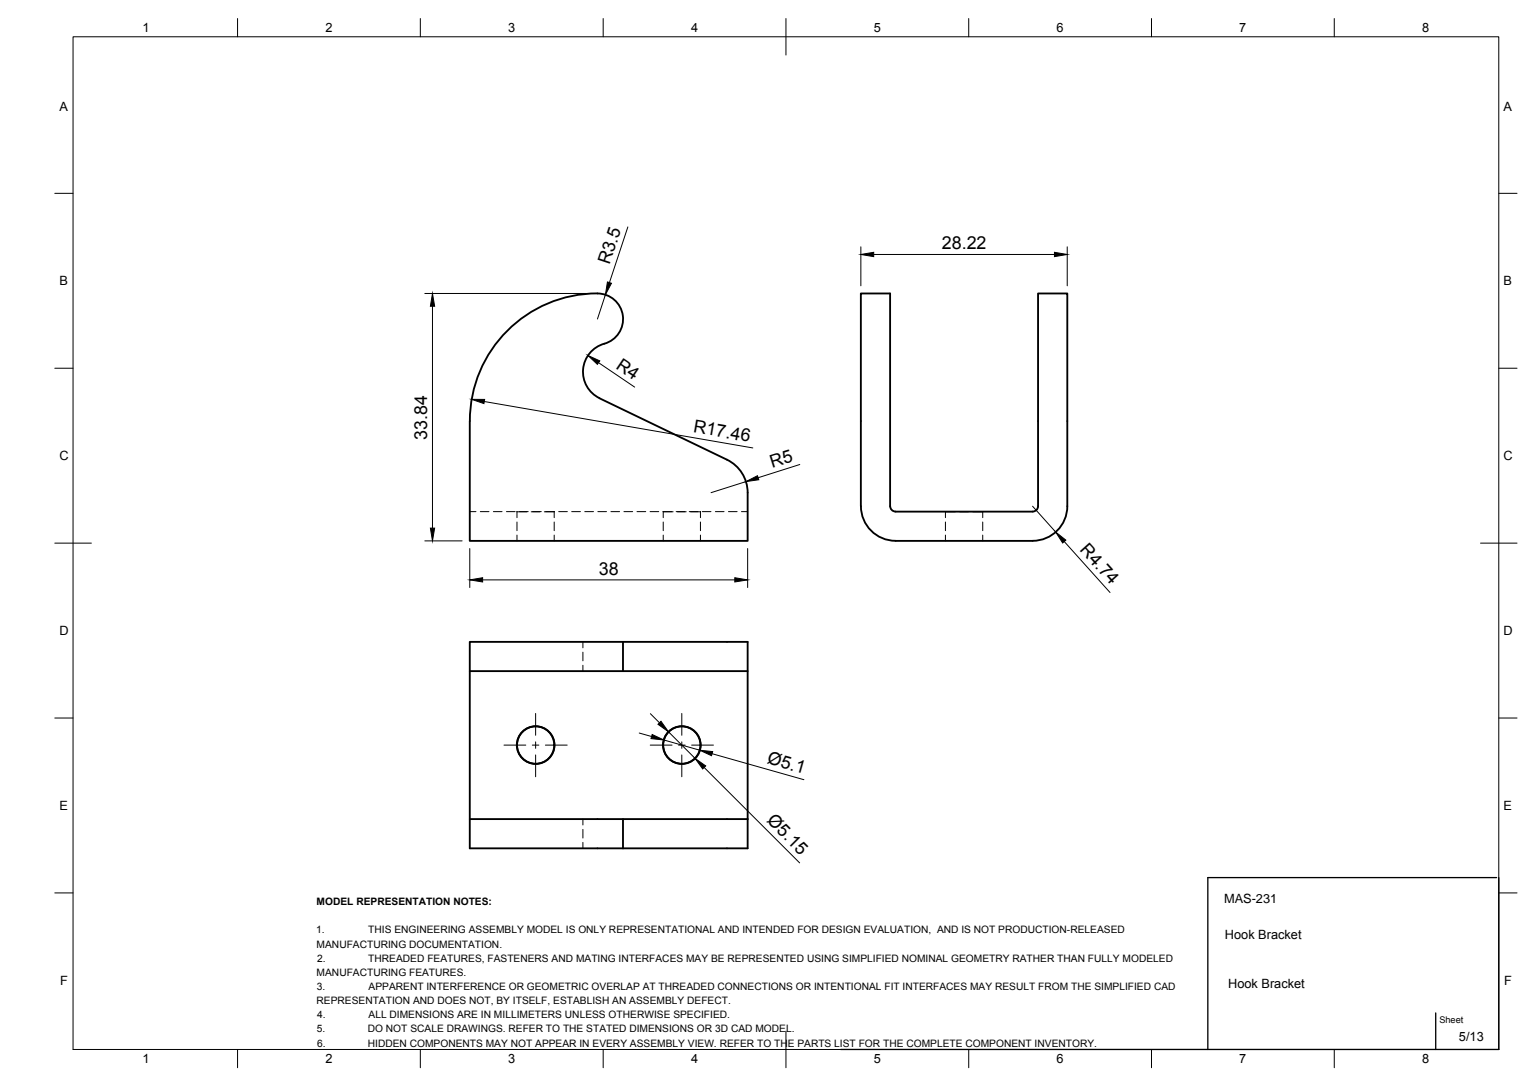
ISO-10303-21;
HEADER;
FILE_DESCRIPTION (('STEP AP214'),
    '1' );
FILE_NAME ( 'Hook Bracket.step', '2026-10-04T02:08:54', ( '' ), ( '' ), 'STEP AP214', 'Unspecified', '' );
FILE_SCHEMA (( 'AUTOMOTIVE_DESIGN' ));
ENDSEC;
DATA;
#98=ORIENTED_EDGE ( 'NONE', *, *, #40284, .T. ) ;
#119=EDGE_LOOP ( 'NONE', ( #9384, #25327, #26730, #11644 ) ) ;
#157=VERTEX_POINT ( 'NONE', #7543 ) ;
#241=ORIENTED_EDGE ( 'NONE', *, *, #39973, .T. ) ;
#254=EDGE_CURVE ( 'NONE', #18975, #21109, #11079, .T. ) ;
#326=AXIS2_PLACEMENT_3D ( 'NONE', #47306, #10657, #25265 ) ;
#395=AXIS2_PLACEMENT_3D ( 'NONE', #5918, #35170, #24842 ) ;
#397=CARTESIAN_POINT ( 'NONE',  ( -0.5555748031496061667, 0.1864803149606364951, -0.7480314960629921295 ) ) ;
#449=CIRCLE ( 'NONE', #39490, 0.02900000000000001882 ) ;
#498=CARTESIAN_POINT ( 'NONE',  ( 0.5555748031496077211, 2.215965818540671970E-15, 0.7480314960629921295 ) ) ;
#504=CIRCLE ( 'NONE', #41823, 0.1003937007874011050 ) ;
#509=ORIENTED_EDGE ( 'NONE', *, *, #3081, .F. ) ;
#538=CARTESIAN_POINT ( 'NONE',  ( -0.5555748031496058337, 0.2597269656108975311, 0.7480314960629921295 ) ) ;
#660=AXIS2_PLACEMENT_3D ( 'NONE', #17202, #46421, #20086 ) ;
#686=EDGE_CURVE ( 'NONE', #23816, #39475, #34433, .T. ) ;
#789=DIRECTION ( 'NONE',  ( -0.000000000000000000, 1.000000000000000000, -0.000000000000000000 ) ) ;
#867=CARTESIAN_POINT ( 'NONE',  ( 0.5555748031496089423, 0.3833307086614172743, 0.7480314960629921295 ) ) ;
#931=ORIENTED_EDGE ( 'NONE', *, *, #9551, .T. ) ;
#1004=VERTEX_POINT ( 'NONE', #1577 ) ;
#1044=CARTESIAN_POINT ( 'NONE',  ( 1.739107093083948175E-16, 0.1574803149606340824, 0.2923228346456709370 ) ) ;
#1068=DIRECTION ( 'NONE',  ( 1.541976423090495042E-15, 0.4344452574044150306, -0.9006982393225888561 ) ) ;
#1160=ORIENTED_EDGE ( 'NONE', *, *, #40875, .T. ) ;
#1198=EDGE_CURVE ( 'NONE', #23361, #25294, #34801, .T. ) ;
#1237=ORIENTED_EDGE ( 'NONE', *, *, #25095, .T. ) ;
#1310=DIRECTION ( 'NONE',  ( -1.000000000000000000, 3.469446951953613794E-15, 0.000000000000000000 ) ) ;
#1348=DIRECTION ( 'NONE',  ( 1.000000000000000000, -3.469446951953613794E-15, -0.000000000000000000 ) ) ;
#1499=CARTESIAN_POINT ( 'NONE',  ( -0.3980944881889741382, 0.7681739484881660029, -0.04983111751016756213 ) ) ;
#1514=FACE_OUTER_BOUND ( 'NONE', #43262, .T. ) ;
#1557=DIRECTION ( 'NONE',  ( 1.000000000000000000, -3.469446951953613794E-15, -0.000000000000000000 ) ) ;
#1577=CARTESIAN_POINT ( 'NONE',  ( 1.614954907737318939E-16, 0.1574803149606340824, 0.4950787401574787139 ) ) ;
#1587=DIRECTION ( 'NONE',  ( 0.000000000000000000, -1.000000000000000000, 0.000000000000000000 ) ) ;
#1618=CARTESIAN_POINT ( 'NONE',  ( -7.957671378281915615E-17, 0.1574803149606340824, -0.2923228346456709370 ) ) ;
#1725=CARTESIAN_POINT ( 'NONE',  ( 0.3980944881889779130, 0.4370297686271517601, 0.6367018223237037589 ) ) ;
#1755=ORIENTED_EDGE ( 'NONE', *, *, #21966, .F. ) ;
#1809=EDGE_CURVE ( 'NONE', #39475, #34571, #39007, .T. ) ;
#1956=EDGE_LOOP ( 'NONE', ( #15134, #37598, #45628, #21040 ) ) ;
#1983=DIMENSIONAL_EXPONENTS ( 1.000000000000000000, 0.000000000000000000, 0.000000000000000000, 0.000000000000000000, 0.000000000000000000, 0.000000000000000000, 0.000000000000000000 ) ;
#2019=VERTEX_POINT ( 'NONE', #7328 ) ;
#2094=VECTOR ( 'NONE', #47331, 39.37007874015748854 ) ;
#2109=EDGE_CURVE ( 'NONE', #33977, #31956, #23129, .T. ) ;
#2130=ORIENTED_EDGE ( 'NONE', *, *, #32542, .F. ) ;
#2161=VECTOR ( 'NONE', #24206, 39.37007874015748143 ) ;
#2318=ADVANCED_FACE ( 'NONE', ( #29029 ), #46707, .T. ) ;
#2362=LINE ( 'NONE', #45498, #19120 ) ;
#2457=LINE ( 'NONE', #17083, #4486 ) ;
#2474=CARTESIAN_POINT ( 'NONE',  ( 0.3690944881889770546, 0.1574803149606328057, 0.7480314960629921295 ) ) ;
#2489=CYLINDRICAL_SURFACE ( 'NONE', #43547, 0.1377952755905521298 ) ;
#2593=AXIS2_PLACEMENT_3D ( 'NONE', #22968, #30429, #44981 ) ;
#2608=CARTESIAN_POINT ( 'NONE',  ( 0.5555748031496109407, 0.9100161909011688088, 0.01858545845903165558 ) ) ;
#2676=AXIS2_PLACEMENT_3D ( 'NONE', #36439, #10566, #40228 ) ;
#2701=FACE_OUTER_BOUND ( 'NONE', #16952, .T. ) ;
#2719=DIRECTION ( 'NONE',  ( -3.469446951953590129E-15, -1.000000000000000000, 0.000000000000000000 ) ) ;
#2727=FACE_OUTER_BOUND ( 'NONE', #31753, .T. ) ;
#2790=ORIENTED_EDGE ( 'NONE', *, *, #43590, .F. ) ;
#2886=ORIENTED_EDGE ( 'NONE', *, *, #14250, .T. ) ;
#2896=CARTESIAN_POINT ( 'NONE',  ( 0.5555748031496123840, 1.332209862199691397, -0.06082000038405670217 ) ) ;
#2949=DIRECTION ( 'NONE',  ( -0.000000000000000000, 1.000000000000000000, -0.000000000000000000 ) ) ;
#2984=EDGE_LOOP ( 'NONE', ( #4268, #8274, #16882, #28951, #15427, #2790, #46729, #33220 ) ) ;
#2993=EDGE_LOOP ( 'NONE', ( #6858, #21214, #41669, #27403 ) ) ;
#3042=CYLINDRICAL_SURFACE ( 'NONE', #26195, 0.1574803149606291142 ) ;
#3075=DIRECTION ( 'NONE',  ( 3.469446951953613794E-15, 1.000000000000000000, 0.000000000000000000 ) ) ;
#3081=EDGE_CURVE ( 'NONE', #34571, #38848, #8006, .T. ) ;
#3137=ORIENTED_EDGE ( 'NONE', *, *, #14250, .F. ) ;
#3165=VERTEX_POINT ( 'NONE', #10746 ) ;
#3205=FACE_OUTER_BOUND ( 'NONE', #16925, .T. ) ;
#3330=LINE ( 'NONE', #32591, #23506 ) ;
#3413=DIRECTION ( 'NONE',  ( 0.000000000000000000, 0.000000000000000000, -1.000000000000000000 ) ) ;
#3478=CARTESIAN_POINT ( 'NONE',  ( -0.5555748031496040573, 0.7681739484881665581, -0.04983111751016756213 ) ) ;
#3650=CARTESIAN_POINT ( 'NONE',  ( -0.3690944881889761664, 0.1574803149606353592, -0.7480314960629921295 ) ) ;
#3686=EDGE_CURVE ( 'NONE', #1004, #10953, #29361, .T. ) ;
#3744=AXIS2_PLACEMENT_3D ( 'NONE', #44263, #36406, #11461 ) ;
#3773=AXIS2_PLACEMENT_3D ( 'NONE', #35805, #2949, #32229 ) ;
#3778=VECTOR ( 'NONE', #30865, 39.37007874015748143 ) ;
#3862=MANIFOLD_SOLID_BREP ( 'Hook Bracket', #17070 ) ;
#3897=VECTOR ( 'NONE', #44937, 39.37007874015748854 ) ;
#3983=ADVANCED_FACE ( 'NONE', ( #13018 ), #33958, .T. ) ;
#4077=VERTEX_POINT ( 'NONE', #5814 ) ;
#4089=VECTOR ( 'NONE', #22486, 39.37007874015748143 ) ;
#4198=LINE ( 'NONE', #30373, #20248 ) ;
#4268=ORIENTED_EDGE ( 'NONE', *, *, #43106, .F. ) ;
#4318=CARTESIAN_POINT ( 'NONE',  ( 1.614954907737318939E-16, 0.1574803149606340824, 0.3937007874015748254 ) ) ;
#4360=ORIENTED_EDGE ( 'NONE', *, *, #40924, .F. ) ;
#4390=AXIS2_PLACEMENT_3D ( 'NONE', #10675, #40108, #14018 ) ;
#4486=VECTOR ( 'NONE', #16161, 39.37007874015748143 ) ;
#4561=ORIENTED_EDGE ( 'NONE', *, *, #23328, .T. ) ;
#4584=ORIENTED_EDGE ( 'NONE', *, *, #32997, .F. ) ;
#4633=AXIS2_PLACEMENT_3D ( 'NONE', #24573, #6345, #46368 ) ;
#4691=ADVANCED_FACE ( 'NONE', ( #21545, #20835, #17017 ), #27840, .T. ) ;
#4789=CIRCLE ( 'NONE', #46111, 0.1574803149606301966 ) ;
#4839=FACE_OUTER_BOUND ( 'NONE', #33641, .T. ) ;
#4908=FACE_OUTER_BOUND ( 'NONE', #46312, .T. ) ;
#4919=VECTOR ( 'NONE', #1557, 39.37007874015748143 ) ;
#4975=EDGE_CURVE ( 'NONE', #11301, #39475, #11250, .T. ) ;
#5022=AXIS2_PLACEMENT_3D ( 'NONE', #20568, #24186, #12707 ) ;
#5025=DIRECTION ( 'NONE',  ( -3.469446951953613794E-15, -1.000000000000000000, 0.000000000000000000 ) ) ;
#5134=EDGE_LOOP ( 'NONE', ( #14252, #38748, #44441, #32739, #28557, #35520, #1237, #38379, #3137, #241, #10330, #17989 ) ) ;
#5307=AXIS2_PLACEMENT_3D ( 'NONE', #24089, #24779, #39377 ) ;
#5350=FACE_OUTER_BOUND ( 'NONE', #46134, .T. ) ;
#5405=FACE_BOUND ( 'NONE', #26025, .T. ) ;
#5450=ORIENTED_EDGE ( 'NONE', *, *, #32997, .T. ) ;
#5466=ORIENTED_EDGE ( 'NONE', *, *, #16551, .T. ) ;
#5487=VECTOR ( 'NONE', #17364, 39.37007874015748854 ) ;
#5632=ORIENTED_EDGE ( 'NONE', *, *, #3686, .F. ) ;
#5727=UNCERTAINTY_MEASURE_WITH_UNIT (LENGTH_MEASURE( 1.000000000000000082E-05 ), #6167, 'distance_accuracy_value', 'NONE') ;
#5755=AXIS2_PLACEMENT_3D ( 'NONE', #8382, #41424, #22289 ) ;
#5756=ADVANCED_FACE ( 'NONE', ( #12240 ), #12007, .T. ) ;
#5783=DIRECTION ( 'NONE',  ( 0.000000000000000000, 0.7071067811865965336, 0.7071067811864983899 ) ) ;
#5814=CARTESIAN_POINT ( 'NONE',  ( 0.5555748031496103856, 0.7681739484881628943, -0.04983111751016747887 ) ) ;
#5816=CIRCLE ( 'NONE', #35657, 0.6872114956789353579 ) ;
#5832=DIRECTION ( 'NONE',  ( 3.469446951953626022E-15, 1.000000000000000000, 0.000000000000000000 ) ) ;
#5918=CARTESIAN_POINT ( 'NONE',  ( -0.3690944881889761109, 0.1864803149606353017, 0.7480314960629921295 ) ) ;
#5990=CARTESIAN_POINT ( 'NONE',  ( -0.5555748031496045014, 0.6449983665207589256, -0.7480314960629921295 ) ) ;
#5993=VERTEX_POINT ( 'NONE', #29714 ) ;
#6018=ORIENTED_EDGE ( 'NONE', *, *, #41186, .F. ) ;
#6167=( CONVERSION_BASED_UNIT ( 'INCH', #39466 ) LENGTH_UNIT ( ) NAMED_UNIT ( #22776 ) ) ;
#6188=AXIS2_PLACEMENT_3D ( 'NONE', #9502, #46136, #27264 ) ;
#6251=ORIENTED_EDGE ( 'NONE', *, *, #19100, .T. ) ;
#6325=CARTESIAN_POINT ( 'NONE',  ( 0.3980944881889795228, 0.9100161909011693639, 0.01858545845903165558 ) ) ;
#6345=DIRECTION ( 'NONE',  ( -3.469446951953613794E-15, -1.000000000000000000, 0.000000000000000000 ) ) ;
#6347=CARTESIAN_POINT ( 'NONE',  ( 0.3690944881889778317, 2.862949378880179425E-15, 0.7480314960629921295 ) ) ;
#6355=CARTESIAN_POINT ( 'NONE',  ( -0.3690944881889761109, 0.1864803149606354127, 0.7480314960629921295 ) ) ;
#6360=ORIENTED_EDGE ( 'NONE', *, *, #11275, .F. ) ;
#6368=ADVANCED_FACE ( 'NONE', ( #4908 ), #46344, .F. ) ;
#6376=CARTESIAN_POINT ( 'NONE',  ( 1.737901732061166719E-16, 0.1564960629921311464, 0.2933070866141737065 ) ) ;
#6390=PRODUCT_DEFINITION ( 'UNKNOWN', '', #25524, #46091 ) ;
#6407=CARTESIAN_POINT ( 'NONE',  ( 0.5555748031496109407, 0.9100161909011688088, 0.01858545845903165558 ) ) ;
#6460=DIRECTION ( 'NONE',  ( 3.385139170096243171E-15, 1.000000000000000000, -0.000000000000000000 ) ) ;
#6558=CIRCLE ( 'NONE', #5022, 0.1003937007874011050 ) ;
#6641=FILL_AREA_STYLE_COLOUR ( '', #45353 ) ;
#6647=ORIENTED_EDGE ( 'NONE', *, *, #1809, .F. ) ;
#6682=DIRECTION ( 'NONE',  ( -3.469446951953613794E-15, -1.000000000000000000, -3.652049423109077687E-16 ) ) ;
#6742=( NAMED_UNIT ( * ) PLANE_ANGLE_UNIT ( ) SI_UNIT ( $, .RADIAN. ) ) ;
#6852=AXIS2_PLACEMENT_3D ( 'NONE', #10460, #31568, #14289 ) ;
#6858=ORIENTED_EDGE ( 'NONE', *, *, #12795, .F. ) ;
#6910=DIRECTION ( 'NONE',  ( 1.000000000000000000, -3.469446951953625233E-15, -0.000000000000000000 ) ) ;
#6936=EDGE_CURVE ( 'NONE', #13381, #27058, #4198, .T. ) ;
#6946=VECTOR ( 'NONE', #24006, 39.37007874015748143 ) ;
#7158=CARTESIAN_POINT ( 'NONE',  ( 0.5555748031496118289, 1.194414586609139128, -0.06082000038405787484 ) ) ;
#7197=VECTOR ( 'NONE', #26346, 39.37007874015748143 ) ;
#7244=FACE_OUTER_BOUND ( 'NONE', #5134, .T. ) ;
#7309=DIRECTION ( 'NONE',  ( -3.494233027178502331E-15, -1.000000000000000000, -0.000000000000000000 ) ) ;
#7328=CARTESIAN_POINT ( 'NONE',  ( -0.3690944881889767215, 5.970426471673286898E-15, -0.7480314960629921295 ) ) ;
#7332=ORIENTED_EDGE ( 'NONE', *, *, #16551, .F. ) ;
#7393=FACE_OUTER_BOUND ( 'NONE', #39319, .T. ) ;
#7416=ADVANCED_FACE ( 'NONE', ( #3205 ), #43453, .T. ) ;
#7428=ORIENTED_EDGE ( 'NONE', *, *, #45869, .F. ) ;
#7447=ORIENTED_EDGE ( 'NONE', *, *, #11487, .T. ) ;
#7543=CARTESIAN_POINT ( 'NONE',  ( 0.5555748031496099415, 0.6449983665207553729, -0.7480314960629920185 ) ) ;
#7566=ORIENTED_EDGE ( 'NONE', *, *, #9639, .F. ) ;
#7618=EDGE_CURVE ( 'NONE', #31956, #27577, #33425, .T. ) ;
#7621=ORIENTED_EDGE ( 'NONE', *, *, #13429, .T. ) ;
#7636=ORIENTED_EDGE ( 'NONE', *, *, #39035, .F. ) ;
#7689=SHAPE_REPRESENTATION_RELATIONSHIP ( 'NONE' , 'NONE' ,  #11151, #38737 ) ;
#7744=VERTEX_POINT ( 'NONE', #37865 ) ;
#7760=AXIS2_PLACEMENT_3D ( 'NONE', #42762, #35155, #1587 ) ;
#7773=ORIENTED_EDGE ( 'NONE', *, *, #43106, .T. ) ;
#7870=DIRECTION ( 'NONE',  ( -0.000000000000000000, 1.000000000000000000, -0.000000000000000000 ) ) ;
#7887=ORIENTED_EDGE ( 'NONE', *, *, #30299, .F. ) ;
#7975=AXIS2_PLACEMENT_3D ( 'NONE', #31654, #6682, #13888 ) ;
#7999=VECTOR ( 'NONE', #10189, 39.37007874015748143 ) ;
#8006=LINE ( 'NONE', #11627, #22275 ) ;
#8107=CARTESIAN_POINT ( 'NONE',  ( 0.5555748031496077211, 2.215965818540671970E-15, 0.7480314960629921295 ) ) ;
#8274=ORIENTED_EDGE ( 'NONE', *, *, #16350, .T. ) ;
#8355=CARTESIAN_POINT ( 'NONE',  ( -0.5555748031496021699, 1.332209862199694284, -0.06082000038405668829 ) ) ;
#8382=CARTESIAN_POINT ( 'NONE',  ( -0.3690944881889761109, 0.1864803149606356070, -0.06082000038405686176 ) ) ;
#8408=CARTESIAN_POINT ( 'NONE',  ( -6.728203135043436585E-17, -8.878505979408855953E-16, -0.4940944881889759444 ) ) ;
#8483=ORIENTED_EDGE ( 'NONE', *, *, #21818, .T. ) ;
#8491=CARTESIAN_POINT ( 'NONE',  ( -0.3980944881889759146, 0.2597269656108969760, 0.5511811023622046335 ) ) ;
#8503=ORIENTED_EDGE ( 'NONE', *, *, #30299, .T. ) ;
#8510=ORIENTED_EDGE ( 'NONE', *, *, #37835, .T. ) ;
#8584=APPLICATION_CONTEXT ( 'automotive_design' ) ;
#8604=ADVANCED_FACE ( 'NONE', ( #30707 ), #27119, .F. ) ;
#8676=VECTOR ( 'NONE', #6460, 39.37007874015748143 ) ;
#8731=CARTESIAN_POINT ( 'NONE',  ( 0.5555748031496083872, 0.1864803149606326926, -0.7480314960629921295 ) ) ;
#8737=CARTESIAN_POINT ( 'NONE',  ( -0.3980944881889755260, 0.3833307086614208270, 0.7480314960629921295 ) ) ;
#8832=DIRECTION ( 'NONE',  ( -3.469446951953613794E-15, -1.000000000000000000, 0.000000000000000000 ) ) ;
#8892=ORIENTED_EDGE ( 'NONE', *, *, #30656, .T. ) ;
#8924=DIRECTION ( 'NONE',  ( 0.000000000000000000, 1.000000000000000000, 0.000000000000000000 ) ) ;
#9004=CARTESIAN_POINT ( 'NONE',  ( -0.5555748031496040573, 0.7681739484881661140, -0.04983111751016786051 ) ) ;
#9056=CARTESIAN_POINT ( 'NONE',  ( -0.5555748031496045014, 0.6449983665207589256, -0.06082000038405668829 ) ) ;
#9100=EDGE_CURVE ( 'NONE', #14069, #33762, #27232, .T. ) ;
#9272=CYLINDRICAL_SURFACE ( 'NONE', #7760, 0.1864803149606299171 ) ;
#9280=ORIENTED_EDGE ( 'NONE', *, *, #28375, .F. ) ;
#9338=ORIENTED_EDGE ( 'NONE', *, *, #14169, .T. ) ;
#9384=ORIENTED_EDGE ( 'NONE', *, *, #43378, .T. ) ;
#9400=AXIS2_PLACEMENT_3D ( 'NONE', #4318, #8832, #12694 ) ;
#9464=VERTEX_POINT ( 'NONE', #16370 ) ;
#9479=VERTEX_POINT ( 'NONE', #1725 ) ;
#9502=CARTESIAN_POINT ( 'NONE',  ( -0.3980944881889745268, 0.6449983665207583705, -0.06082000038405668829 ) ) ;
#9523=DIRECTION ( 'NONE',  ( 1.000000000000000000, -3.469446951953614189E-15, -0.000000000000000000 ) ) ;
#9551=EDGE_CURVE ( 'NONE', #19046, #2019, #3330, .T. ) ;
#9554=SURFACE_STYLE_FILL_AREA ( #28238 ) ;
#9587=LINE ( 'NONE', #9824, #2161 ) ;
#9628=DIRECTION ( 'NONE',  ( 3.469446951953608272E-15, 1.000000000000000000, 0.000000000000000000 ) ) ;
#9639=EDGE_CURVE ( 'NONE', #35496, #36366, #504, .T. ) ;
#9692=FACE_OUTER_BOUND ( 'NONE', #1956, .T. ) ;
#9714=CYLINDRICAL_SURFACE ( 'NONE', #17689, 0.02900000000000001882 ) ;
#9738=ORIENTED_EDGE ( 'NONE', *, *, #31992, .T. ) ;
#9757=ADVANCED_FACE ( 'NONE', ( #4839 ), #12039, .F. ) ;
#9807=CIRCLE ( 'NONE', #4390, 0.1003937007874011050 ) ;
#9824=CARTESIAN_POINT ( 'NONE',  ( 1.737901732061166719E-16, 0.1574803149606340824, 0.2933070866141737065 ) ) ;
#9915=VECTOR ( 'NONE', #5783, 39.37007874015748854 ) ;
#9937=DIRECTION ( 'NONE',  ( -1.000000000000000000, 3.469446951953614189E-15, 0.000000000000000000 ) ) ;
#9969=ADVANCED_FACE ( 'NONE', ( #2701 ), #13973, .F. ) ;
#10002=VECTOR ( 'NONE', #1068, 39.37007874015748854 ) ;
#10051=DIRECTION ( 'NONE',  ( 1.000000000000000000, 0.000000000000000000, 0.000000000000000000 ) ) ;
#10104=AXIS2_PLACEMENT_3D ( 'NONE', #15674, #44861, #30080 ) ;
#10189=DIRECTION ( 'NONE',  ( -1.000000000000000000, 3.469446951953613794E-15, 0.000000000000000000 ) ) ;
#10222=VERTEX_POINT ( 'NONE', #38556 ) ;
#10257=CARTESIAN_POINT ( 'NONE',  ( -0.3690944881889761109, 0.1864803149606358568, -0.7480314960629921295 ) ) ;
#10301=ORIENTED_EDGE ( 'NONE', *, *, #45389, .F. ) ;
#10330=ORIENTED_EDGE ( 'NONE', *, *, #30656, .F. ) ;
#10333=ORIENTED_EDGE ( 'NONE', *, *, #16196, .F. ) ;
#10337=CONICAL_SURFACE ( 'NONE', #34066, 0.1003937007874011050, 0.7853981633973787790 ) ;
#10460=CARTESIAN_POINT ( 'NONE',  ( 0.3690944881889771101, 0.1864803149606328037, -0.7480314960629921295 ) ) ;
#10480=ORIENTED_EDGE ( 'NONE', *, *, #19100, .F. ) ;
#10566=DIRECTION ( 'NONE',  ( -0.000000000000000000, 1.000000000000000000, -0.000000000000000000 ) ) ;
#10657=DIRECTION ( 'NONE',  ( -1.000000000000000000, 3.469446951953614189E-15, 0.000000000000000000 ) ) ;
#10667=CARTESIAN_POINT ( 'NONE',  ( 0.3980944881889786346, 0.6449983665207558170, -0.06082000038405668829 ) ) ;
#10675=CARTESIAN_POINT ( 'NONE',  ( 1.614954907737318939E-16, 0.1564960629921311464, 0.3937007874015748254 ) ) ;
#10696=DIRECTION ( 'NONE',  ( 1.000000000000000000, 0.000000000000000000, 0.000000000000000000 ) ) ;
#10743=DIRECTION ( 'NONE',  ( -1.000000000000000000, 0.000000000000000000, 0.000000000000000000 ) ) ;
#10746=CARTESIAN_POINT ( 'NONE',  ( 0.5555748031496114958, 1.061695335278752150, -0.02376411959061622975 ) ) ;
#10747=AXIS2_PLACEMENT_3D ( 'NONE', #29942, #22224, #33053 ) ;
#10835=DIRECTION ( 'NONE',  ( 1.000000000000000000, 0.000000000000000000, 0.000000000000000000 ) ) ;
#10842=EDGE_CURVE ( 'NONE', #7744, #18975, #47081, .T. ) ;
#10953=VERTEX_POINT ( 'NONE', #1044 ) ;
#10960=EDGE_CURVE ( 'NONE', #4077, #14069, #34374, .T. ) ;
#11079=CIRCLE ( 'NONE', #27928, 0.1574803149606301966 ) ;
#11147=CARTESIAN_POINT ( 'NONE',  ( 0.5555748031496083872, 0.1864803149606321375, 0.7480314960629921295 ) ) ;
#11151=SHAPE_REPRESENTATION ( 'Hook Bracket', ( #20860 ), #31601 ) ;
#11183=AXIS2_PLACEMENT_3D ( 'NONE', #42840, #14124, #10051 ) ;
#11195=ORIENTED_EDGE ( 'NONE', *, *, #10842, .F. ) ;
#11250=LINE ( 'NONE', #29964, #7197 ) ;
#11253=LINE ( 'NONE', #8107, #4089 ) ;
#11275=EDGE_CURVE ( 'NONE', #21453, #25294, #22792, .T. ) ;
#11301=VERTEX_POINT ( 'NONE', #2474 ) ;
#11352=ORIENTED_EDGE ( 'NONE', *, *, #43378, .F. ) ;
#11388=VERTEX_POINT ( 'NONE', #17338 ) ;
#11403=EDGE_LOOP ( 'NONE', ( #35721, #31288, #38159, #34983 ) ) ;
#11461=DIRECTION ( 'NONE',  ( 3.469446951953620894E-15, 1.000000000000000000, 0.000000000000000000 ) ) ;
#11487=EDGE_CURVE ( 'NONE', #16814, #23361, #43909, .T. ) ;
#11493=DIRECTION ( 'NONE',  ( -0.000000000000000000, -0.000000000000000000, 1.000000000000000000 ) ) ;
#11520=AXIS2_PLACEMENT_3D ( 'NONE', #27824, #5025, #42384 ) ;
#11538=VECTOR ( 'NONE', #14914, 39.37007874015748143 ) ;
#11627=CARTESIAN_POINT ( 'NONE',  ( 0.3980944881889770248, 0.1864803149606327204, 0.7480314960629921295 ) ) ;
#11639=DIRECTION ( 'NONE',  ( 1.000000000000000000, -3.469446951953626022E-15, -0.000000000000000000 ) ) ;
#11644=ORIENTED_EDGE ( 'NONE', *, *, #31492, .T. ) ;
#11658=CARTESIAN_POINT ( 'NONE',  ( -7.957671378281915615E-17, 0.1574803149606340824, -0.3937007874015748254 ) ) ;
#11671=CARTESIAN_POINT ( 'NONE',  ( -0.5555748031496060557, 0.1864803149606359678, 0.7480314960629921295 ) ) ;
#11730=CARTESIAN_POINT ( 'NONE',  ( -6.728203135043436585E-17, 0.1574803149606340824, -0.4940944881889759444 ) ) ;
#11858=DIRECTION ( 'NONE',  ( -1.000000000000000000, 3.469446951953613794E-15, 0.000000000000000000 ) ) ;
#11916=CARTESIAN_POINT ( 'NONE',  ( -0.3980944881889759146, 0.2597269656108969760, 0.7480314960629921295 ) ) ;
#11932=CARTESIAN_POINT ( 'NONE',  ( -0.3690944881889761109, 0.1864803149606354127, -0.7480314960629921295 ) ) ;
#11961=EDGE_LOOP ( 'NONE', ( #12897, #26559, #41039, #33100, #35426, #8503, #41723, #31883, #46859, #7428, #25835, #98 ) ) ;
#12007=CYLINDRICAL_SURFACE ( 'NONE', #5755, 0.1864803149606298893 ) ;
#12039=CONICAL_SURFACE ( 'NONE', #40325, 0.1003937007874011050, 0.7853981633973787790 ) ;
#12117=ORIENTED_EDGE ( 'NONE', *, *, #3081, .T. ) ;
#12162=DIRECTION ( 'NONE',  ( 3.124924761047742408E-15, 0.9006982393225889671, 0.4344452574044149751 ) ) ;
#12240=FACE_OUTER_BOUND ( 'NONE', #21625, .T. ) ;
#12271=CIRCLE ( 'NONE', #10747, 0.1968503937007874127 ) ;
#12280=AXIS2_PLACEMENT_3D ( 'NONE', #13897, #43109, #24926 ) ;
#12349=CARTESIAN_POINT ( 'NONE',  ( -0.5555748031496036132, 0.9100161909011723615, 0.01858545845903165558 ) ) ;
#12593=DIRECTION ( 'NONE',  ( -3.469446951953608272E-15, -1.000000000000000000, 0.000000000000000000 ) ) ;
#12673=CIRCLE ( 'NONE', #2676, 0.1003937007874011050 ) ;
#12678=CIRCLE ( 'NONE', #395, 0.1864803149606299171 ) ;
#12694=DIRECTION ( 'NONE',  ( 1.000000000000000000, -3.368395098984144529E-15, 0.000000000000000000 ) ) ;
#12707=DIRECTION ( 'NONE',  ( 0.000000000000000000, 0.000000000000000000, -1.000000000000000000 ) ) ;
#12714=ORIENTED_EDGE ( 'NONE', *, *, #10960, .T. ) ;
#12795=EDGE_CURVE ( 'NONE', #10222, #35496, #9587, .T. ) ;
#12806=ORIENTED_EDGE ( 'NONE', *, *, #9100, .F. ) ;
#12811=CARTESIAN_POINT ( 'NONE',  ( 1.614954907737318939E-16, 0.1574803149606340824, 0.4940944881889759444 ) ) ;
#12891=DIRECTION ( 'NONE',  ( 3.469446951953614189E-15, 1.000000000000000000, 0.000000000000000000 ) ) ;
#12897=ORIENTED_EDGE ( 'NONE', *, *, #13858, .T. ) ;
#12939=CIRCLE ( 'NONE', #3744, 0.1377952755905509086 ) ;
#12960=EDGE_CURVE ( 'NONE', #21109, #22330, #12939, .T. ) ;
#13018=FACE_OUTER_BOUND ( 'NONE', #11961, .T. ) ;
#13070=ADVANCED_FACE ( 'NONE', ( #7393 ), #18408, .F. ) ;
#13105=DIRECTION ( 'NONE',  ( -1.000000000000000000, 3.469446951953614189E-15, 0.000000000000000000 ) ) ;
#13135=LINE ( 'NONE', #6376, #32082 ) ;
#13169=CIRCLE ( 'NONE', #39916, 0.1377952755905509086 ) ;
#13183=ORIENTED_EDGE ( 'NONE', *, *, #44180, .F. ) ;
#13303=FACE_OUTER_BOUND ( 'NONE', #20319, .T. ) ;
#13329=DIRECTION ( 'NONE',  ( -3.469446951953590129E-15, -1.000000000000000000, 0.000000000000000000 ) ) ;
#13371=DIRECTION ( 'NONE',  ( -1.000000000000000000, 3.469446951953626022E-15, 0.000000000000000000 ) ) ;
#13381=VERTEX_POINT ( 'NONE', #31579 ) ;
#13425=AXIS2_PLACEMENT_3D ( 'NONE', #26632, #37152, #41184 ) ;
#13429=EDGE_CURVE ( 'NONE', #35496, #10953, #13135, .T. ) ;
#13486=ADVANCED_FACE ( 'NONE', ( #39908 ), #26030, .F. ) ;
#13513=DIRECTION ( 'NONE',  ( -3.469446951953613794E-15, -1.000000000000000000, 0.000000000000000000 ) ) ;
#13531=CARTESIAN_POINT ( 'NONE',  ( 0.5555748031496099415, 0.6449983665207553729, -0.7480314960629920185 ) ) ;
#13585=CARTESIAN_POINT ( 'NONE',  ( 1.614954907737318939E-16, -8.878505979408855953E-16, 0.4940944881889759444 ) ) ;
#13618=VECTOR ( 'NONE', #23347, 39.37007874015748143 ) ;
#13702=DIRECTION ( 'NONE',  ( -1.000000000000000000, 3.469446951953613794E-15, 0.000000000000000000 ) ) ;
#13743=CARTESIAN_POINT ( 'NONE',  ( -0.5555748031496058337, 0.2597269656108975311, 0.5511811023622046335 ) ) ;
#13763=FACE_OUTER_BOUND ( 'NONE', #30767, .T. ) ;
#13839=( NAMED_UNIT ( * ) SI_UNIT ( $, .STERADIAN. ) SOLID_ANGLE_UNIT ( ) ) ;
#13858=EDGE_CURVE ( 'NONE', #40321, #2019, #34181, .T. ) ;
#13888=DIRECTION ( 'NONE',  ( 1.000000000000000000, -3.469446951953613794E-15, 0.000000000000000000 ) ) ;
#13897=CARTESIAN_POINT ( 'NONE',  ( -0.5555748031496026140, 1.194414586609142903, -0.06082000038405787484 ) ) ;
#13973=CYLINDRICAL_SURFACE ( 'NONE', #30426, 0.02900000000000001882 ) ;
#14018=DIRECTION ( 'NONE',  ( 0.000000000000000000, 0.000000000000000000, -1.000000000000000000 ) ) ;
#14027=CARTESIAN_POINT ( 'NONE',  ( -0.3980944881889761366, 0.1864803149606355515, -0.06082000038405668829 ) ) ;
#14068=ADVANCED_FACE ( 'NONE', ( #13303 ), #2489, .T. ) ;
#14069=VERTEX_POINT ( 'NONE', #38698 ) ;
#14086=PRESENTATION_STYLE_ASSIGNMENT (( #46895 ) ) ;
#14092=CARTESIAN_POINT ( 'NONE',  ( 0.3980944881889800779, 1.061695335278752594, -0.02376411959061622975 ) ) ;
#14124=DIRECTION ( 'NONE',  ( 0.000000000000000000, -0.000000000000000000, 1.000000000000000000 ) ) ;
#14144=ADVANCED_FACE ( 'NONE', ( #28159 ), #42963, .F. ) ;
#14169=EDGE_CURVE ( 'NONE', #16814, #33534, #46627, .T. ) ;
#14250=EDGE_CURVE ( 'NONE', #38848, #27058, #25963, .T. ) ;
#14252=ORIENTED_EDGE ( 'NONE', *, *, #2109, .T. ) ;
#14289=DIRECTION ( 'NONE',  ( -1.000000000000000000, -1.177520686924250585E-15, 0.000000000000000000 ) ) ;
#14383=AXIS2_PLACEMENT_3D ( 'NONE', #17366, #42986, #29155 ) ;
#14421=EDGE_LOOP ( 'NONE', ( #12806, #29972, #28451, #5450 ) ) ;
#14458=DIRECTION ( 'NONE',  ( -0.000000000000000000, 1.000000000000000000, -0.000000000000000000 ) ) ;
#14544=AXIS2_PLACEMENT_3D ( 'NONE', #867, #12162, #26788 ) ;
#14596=ORIENTED_EDGE ( 'NONE', *, *, #11487, .F. ) ;
#14757=AXIS2_PLACEMENT_3D ( 'NONE', #20393, #27633, #9628 ) ;
#14776=AXIS2_PLACEMENT_3D ( 'NONE', #33484, #27886, #42447 ) ;
#14777=ORIENTED_EDGE ( 'NONE', *, *, #41186, .T. ) ;
#14824=CARTESIAN_POINT ( 'NONE',  ( 1.614954907737318939E-16, 0.1574803149606340824, 0.3937007874015748254 ) ) ;
#14914=DIRECTION ( 'NONE',  ( 1.000000000000000000, -3.469446951953625233E-15, -0.000000000000000000 ) ) ;
#14945=ORIENTED_EDGE ( 'NONE', *, *, #35872, .F. ) ;
#14999=PRODUCT_DEFINITION_SHAPE ( 'NONE', 'NONE',  #6390 ) ;
#15011=EDGE_LOOP ( 'NONE', ( #38695, #19381, #8892, #42251 ) ) ;
#15134=ORIENTED_EDGE ( 'NONE', *, *, #33690, .F. ) ;
#15209=LINE ( 'NONE', #44635, #34567 ) ;
#15215=AXIS2_PLACEMENT_3D ( 'NONE', #11658, #22417, #28946 ) ;
#15369=ORIENTED_EDGE ( 'NONE', *, *, #21818, .F. ) ;
#15374=CIRCLE ( 'NONE', #29210, 0.1377952755905521298 ) ;
#15391=DIRECTION ( 'NONE',  ( 0.000000000000000000, -0.000000000000000000, 1.000000000000000000 ) ) ;
#15427=ORIENTED_EDGE ( 'NONE', *, *, #40661, .F. ) ;
#15449=CIRCLE ( 'NONE', #10104, 0.1013779527559039162 ) ;
#15450=VECTOR ( 'NONE', #39879, 39.37007874015748143 ) ;
#15466=CARTESIAN_POINT ( 'NONE',  ( -7.957671378281915615E-17, -8.878505979408855953E-16, -0.2933070866141737065 ) ) ;
#15527=FACE_OUTER_BOUND ( 'NONE', #20527, .T. ) ;
#15532=MECHANICAL_DESIGN_GEOMETRIC_PRESENTATION_REPRESENTATION('',(#23184),#18587);
#15623=VECTOR ( 'NONE', #7870, 39.37007874015748143 ) ;
#15674=CARTESIAN_POINT ( 'NONE',  ( 1.614954907737318939E-16, 0.1574803149606340824, 0.3937007874015748254 ) ) ;
#15687=LINE ( 'NONE', #1499, #37080 ) ;
#15828=EDGE_CURVE ( 'NONE', #25294, #21453, #39771, .T. ) ;
#15878=CARTESIAN_POINT ( 'NONE',  ( -0.5555748031496068329, 1.092739197465708640E-15, -0.7480314960629921295 ) ) ;
#15924=FACE_OUTER_BOUND ( 'NONE', #43960, .T. ) ;
#15932=EDGE_CURVE ( 'NONE', #30455, #34571, #2362, .T. ) ;
#15969=ORIENTED_EDGE ( 'NONE', *, *, #39973, .F. ) ;
#15989=LINE ( 'NONE', #30855, #26875 ) ;
#16046=CARTESIAN_POINT ( 'NONE',  ( -0.3690944881889761664, 0.1574803149606353592, -0.7480314960629921295 ) ) ;
#16161=DIRECTION ( 'NONE',  ( 1.000000000000000000, -3.469446951953625233E-15, -2.725366053876155610E-32 ) ) ;
#16196=EDGE_CURVE ( 'NONE', #27058, #9479, #12271, .T. ) ;
#16350=EDGE_CURVE ( 'NONE', #40003, #13381, #18382, .T. ) ;
#16370=CARTESIAN_POINT ( 'NONE',  ( -0.3690944881889761664, 0.1574803149606353592, 0.7480314960629921295 ) ) ;
#16406=ORIENTED_EDGE ( 'NONE', *, *, #40234, .F. ) ;
#16409=ORIENTED_EDGE ( 'NONE', *, *, #11275, .T. ) ;
#16476=ORIENTED_EDGE ( 'NONE', *, *, #26756, .T. ) ;
#16551=EDGE_CURVE ( 'NONE', #9479, #14069, #41539, .T. ) ;
#16731=DIRECTION ( 'NONE',  ( -1.267059173938974432E-30, -3.652049423109077687E-16, 1.000000000000000000 ) ) ;
#16740=DIRECTION ( 'NONE',  ( 1.000000000000000000, -3.469446951953626022E-15, -0.000000000000000000 ) ) ;
#16775=CIRCLE ( 'NONE', #14383, 0.1864803149606299171 ) ;
#16814=VERTEX_POINT ( 'NONE', #15466 ) ;
#16882=ORIENTED_EDGE ( 'NONE', *, *, #25095, .F. ) ;
#16925=EDGE_LOOP ( 'NONE', ( #44590, #6018, #10333, #36513 ) ) ;
#16939=DIRECTION ( 'NONE',  ( 8.659560562354332584E-17, 0.7071067811865965336, -0.7071067811864983899 ) ) ;
#16952=EDGE_LOOP ( 'NONE', ( #7636, #24781, #7887, #15369 ) ) ;
#16960=DIRECTION ( 'NONE',  ( -1.000000000000000000, 3.469446951953614189E-15, 0.000000000000000000 ) ) ;
#17017=FACE_OUTER_BOUND ( 'NONE', #45799, .T. ) ;
#17070=CLOSED_SHELL ( 'NONE', ( #37706, #9757, #13070, #13486, #45875, #21654, #30436, #23277, #4691, #3983, #37501, #14068, #44174, #32110, #23556, #35510, #2318, #26697, #19483, #20289, #8604, #14144, #6368, #19372, #9969, #45786, #5756, #20935, #35023, #7416 ) ) ;
#17083=CARTESIAN_POINT ( 'NONE',  ( -0.3980944881889753040, 0.4370297686271547022, 0.6367018223237037589 ) ) ;
#17135=LINE ( 'NONE', #28415, #5487 ) ;
#17202=CARTESIAN_POINT ( 'NONE',  ( 0.3690944881889771101, 0.1864803149606328037, 0.7480314960629921295 ) ) ;
#17274=CIRCLE ( 'NONE', #23414, 0.6872114956789353579 ) ;
#17320=CARTESIAN_POINT ( 'NONE',  ( -7.957671378281915615E-17, 0.1564960629921311464, -0.3937007874015748254 ) ) ;
#17338=CARTESIAN_POINT ( 'NONE',  ( 0.5555748031496123840, 1.332209862199691397, -0.06082000038405670217 ) ) ;
#17339=CYLINDRICAL_SURFACE ( 'NONE', #42301, 0.1968503937007874127 ) ;
#17356=DIRECTION ( 'NONE',  ( 0.000000000000000000, 0.000000000000000000, 1.000000000000000000 ) ) ;
#17364=DIRECTION ( 'NONE',  ( 8.659560562354332584E-17, 0.7071067811865965336, -0.7071067811864983899 ) ) ;
#17366=CARTESIAN_POINT ( 'NONE',  ( 0.3690944881889784424, 0.1864803149606333310, -0.7480314960629921295 ) ) ;
#17399=EDGE_CURVE ( 'NONE', #36803, #33940, #20152, .T. ) ;
#17431=( LENGTH_UNIT ( ) NAMED_UNIT ( * ) SI_UNIT ( $, .METRE. ) ) ;
#17451=EDGE_LOOP ( 'NONE', ( #22452, #37391, #7447, #42501 ) ) ;
#17468=ORIENTED_EDGE ( 'NONE', *, *, #10842, .T. ) ;
#17522=AXIS2_PLACEMENT_3D ( 'NONE', #14824, #40655, #25385 ) ;
#17670=CARTESIAN_POINT ( 'NONE',  ( -0.3980944881889745268, 0.6449983665207583705, -0.7480314960629921295 ) ) ;
#17689=AXIS2_PLACEMENT_3D ( 'NONE', #38464, #17356, #31531 ) ;
#17773=( NAMED_UNIT ( * ) SI_UNIT ( $, .STERADIAN. ) SOLID_ANGLE_UNIT ( ) ) ;
#17865=DIRECTION ( 'NONE',  ( -0.000000000000000000, 0.000000000000000000, -1.000000000000000000 ) ) ;
#17910=FACE_OUTER_BOUND ( 'NONE', #14421, .T. ) ;
#17951=CIRCLE ( 'NONE', #40106, 0.1003937007874011050 ) ;
#17989=ORIENTED_EDGE ( 'NONE', *, *, #39035, .T. ) ;
#18046=CARTESIAN_POINT ( 'NONE',  ( -7.957671378281915615E-17, 0.1574803149606340824, -0.2933070866141737065 ) ) ;
#18106=ORIENTED_EDGE ( 'NONE', *, *, #3686, .T. ) ;
#18382=CIRCLE ( 'NONE', #45148, 0.1968503937007874127 ) ;
#18408=CYLINDRICAL_SURFACE ( 'NONE', #17522, 0.1003937007874011050 ) ;
#18430=DIRECTION ( 'NONE',  ( 0.000000000000000000, 0.000000000000000000, 1.000000000000000000 ) ) ;
#18494=DIRECTION ( 'NONE',  ( 1.000000000000000000, 0.000000000000000000, -0.000000000000000000 ) ) ;
#18587=( GEOMETRIC_REPRESENTATION_CONTEXT ( 3 ) GLOBAL_UNCERTAINTY_ASSIGNED_CONTEXT ( ( #5727 ) ) GLOBAL_UNIT_ASSIGNED_CONTEXT ( ( #6167, #24630, #13839 ) ) REPRESENTATION_CONTEXT ( 'NONE', 'WORKASPACE' ) ) ;
#18600=EDGE_CURVE ( 'NONE', #2019, #33940, #35337, .T. ) ;
#18780=CARTESIAN_POINT ( 'NONE',  ( -0.3980944881889761366, 0.1864803149606355237, -0.7480314960629921295 ) ) ;
#18823=ORIENTED_EDGE ( 'NONE', *, *, #17399, .T. ) ;
#18839=CIRCLE ( 'NONE', #35587, 0.1377952755905521298 ) ;
#18898=CARTESIAN_POINT ( 'NONE',  ( 1.614954907737318939E-16, -8.878505979408855953E-16, 0.3937007874015748254 ) ) ;
#18899=CARTESIAN_POINT ( 'NONE',  ( -0.3980944881889761922, 0.1864803149606355237, 0.7480314960629921295 ) ) ;
#18948=AXIS2_PLACEMENT_3D ( 'NONE', #23828, #13513, #24305 ) ;
#18975=VERTEX_POINT ( 'NONE', #9004 ) ;
#19046=VERTEX_POINT ( 'NONE', #46593 ) ;
#19100=EDGE_CURVE ( 'NONE', #5993, #21453, #17135, .T. ) ;
#19120=VECTOR ( 'NONE', #23256, 39.37007874015748143 ) ;
#19218=EDGE_CURVE ( 'NONE', #18975, #39762, #15209, .T. ) ;
#19372=ADVANCED_FACE ( 'NONE', ( #31484 ), #29915, .F. ) ;
#19381=ORIENTED_EDGE ( 'NONE', *, *, #37423, .T. ) ;
#19387=DIRECTION ( 'NONE',  ( -1.000000000000000000, 0.000000000000000000, 0.000000000000000000 ) ) ;
#19418=VECTOR ( 'NONE', #11493, 39.37007874015748143 ) ;
#19483=ADVANCED_FACE ( 'NONE', ( #15924 ), #37956, .F. ) ;
#19571=CARTESIAN_POINT ( 'NONE',  ( -0.3980944881889762477, 0.1574803149606354702, -0.7480314960629921295 ) ) ;
#19773=VERTEX_POINT ( 'NONE', #27083 ) ;
#19777=CIRCLE ( 'NONE', #25912, 0.1003937007874011050 ) ;
#19813=CIRCLE ( 'NONE', #660, 0.02900000000000001882 ) ;
#19852=VECTOR ( 'NONE', #1310, 39.37007874015748143 ) ;
#19903=AXIS2_PLACEMENT_3D ( 'NONE', #11932, #44952, #33510 ) ;
#20027=FACE_OUTER_BOUND ( 'NONE', #15011, .T. ) ;
#20039=ORIENTED_EDGE ( 'NONE', *, *, #15828, .F. ) ;
#20044=AXIS2_PLACEMENT_3D ( 'NONE', #21754, #39941, #21501 ) ;
#20086=DIRECTION ( 'NONE',  ( 1.000000000000000000, -3.532562060772751952E-15, 0.000000000000000000 ) ) ;
#20152=LINE ( 'NONE', #15878, #6946 ) ;
#20248=VECTOR ( 'NONE', #44218, 39.37007874015748143 ) ;
#20289=ADVANCED_FACE ( 'NONE', ( #31557 ), #35145, .T. ) ;
#20319=EDGE_LOOP ( 'NONE', ( #38849, #4584, #38629, #36018 ) ) ;
#20393=CARTESIAN_POINT ( 'NONE',  ( -0.5555748031496036132, 0.9100161909011723615, 0.01858545845903165558 ) ) ;
#20448=CARTESIAN_POINT ( 'NONE',  ( -0.5555748031496021699, 1.332209862199694284, -0.06082000038405668829 ) ) ;
#20527=EDGE_LOOP ( 'NONE', ( #7332, #14777, #7773, #12714 ) ) ;
#20568=CARTESIAN_POINT ( 'NONE',  ( -7.957671378281915615E-17, 0.1564960629921311464, -0.3937007874015748254 ) ) ;
#20637=VECTOR ( 'NONE', #30818, 39.37007874015748143 ) ;
#20701=AXIS2_PLACEMENT_3D ( 'NONE', #34605, #23346, #23806 ) ;
#20835=FACE_BOUND ( 'NONE', #24139, .T. ) ;
#20860=AXIS2_PLACEMENT_3D ( 'NONE', #25692, #32652, #10835 ) ;
#20935=ADVANCED_FACE ( 'NONE', ( #42068 ), #9272, .T. ) ;
#20945=DIRECTION ( 'NONE',  ( 3.469446951953613794E-15, 1.000000000000000000, 0.000000000000000000 ) ) ;
#20950=CARTESIAN_POINT ( 'NONE',  ( 0.5555748031496077211, 2.215965818540671970E-15, 0.7480314960629921295 ) ) ;
#21019=DIRECTION ( 'NONE',  ( -1.000000000000000000, 3.469446951953614189E-15, 0.000000000000000000 ) ) ;
#21040=ORIENTED_EDGE ( 'NONE', *, *, #40875, .F. ) ;
#21109=VERTEX_POINT ( 'NONE', #41711 ) ;
#21208=VERTEX_POINT ( 'NONE', #35035 ) ;
#21214=ORIENTED_EDGE ( 'NONE', *, *, #26756, .F. ) ;
#21411=DIRECTION ( 'NONE',  ( 3.385139170096289319E-15, 1.000000000000000000, 0.000000000000000000 ) ) ;
#21453=VERTEX_POINT ( 'NONE', #29309 ) ;
#21501=DIRECTION ( 'NONE',  ( 3.469446951953613794E-15, 1.000000000000000000, 0.000000000000000000 ) ) ;
#21537=ORIENTED_EDGE ( 'NONE', *, *, #40284, .F. ) ;
#21545=FACE_BOUND ( 'NONE', #34728, .T. ) ;
#21625=EDGE_LOOP ( 'NONE', ( #25371, #36176, #32578, #43915 ) ) ;
#21627=DIRECTION ( 'NONE',  ( 0.000000000000000000, 1.000000000000000000, 0.000000000000000000 ) ) ;
#21654=ADVANCED_FACE ( 'NONE', ( #17910 ), #3042, .F. ) ;
#21754=CARTESIAN_POINT ( 'NONE',  ( -0.5555748031496058337, 0.2597269656108975311, 0.5511811023622046335 ) ) ;
#21818=EDGE_CURVE ( 'NONE', #33977, #26206, #31787, .T. ) ;
#21925=PLANE ( 'NONE',  #44579 ) ;
#21943=VERTEX_POINT ( 'NONE', #6347 ) ;
#21966=EDGE_CURVE ( 'NONE', #27280, #26206, #35607, .T. ) ;
#22224=DIRECTION ( 'NONE',  ( -1.000000000000000000, 3.469446951953614189E-15, 0.000000000000000000 ) ) ;
#22230=DIRECTION ( 'NONE',  ( 1.000000000000000000, -3.469446951953614189E-15, -0.000000000000000000 ) ) ;
#22275=VECTOR ( 'NONE', #26246, 39.37007874015748143 ) ;
#22289=DIRECTION ( 'NONE',  ( 0.000000000000000000, 1.000000000000000000, 3.662381193212024518E-16 ) ) ;
#22330=VERTEX_POINT ( 'NONE', #20448 ) ;
#22417=DIRECTION ( 'NONE',  ( -0.000000000000000000, 1.000000000000000000, -0.000000000000000000 ) ) ;
#22423=DIRECTION ( 'NONE',  ( 0.000000000000000000, 0.000000000000000000, 1.000000000000000000 ) ) ;
#22451=PLANE ( 'NONE',  #14544 ) ;
#22452=ORIENTED_EDGE ( 'NONE', *, *, #25107, .F. ) ;
#22478=ORIENTED_EDGE ( 'NONE', *, *, #32542, .T. ) ;
#22486=DIRECTION ( 'NONE',  ( 3.385139170096289319E-15, 1.000000000000000000, 0.000000000000000000 ) ) ;
#22740=LINE ( 'NONE', #16046, #19418 ) ;
#22776=DIMENSIONAL_EXPONENTS ( 1.000000000000000000, 0.000000000000000000, 0.000000000000000000, 0.000000000000000000, 0.000000000000000000, 0.000000000000000000, 0.000000000000000000 ) ;
#22792=CIRCLE ( 'NONE', #18948, 0.1013779527559039162 ) ;
#22968=CARTESIAN_POINT ( 'NONE',  ( 0.5555748031496109407, 0.9100161909011688088, 0.01858545845903165558 ) ) ;
#22996=ORIENTED_EDGE ( 'NONE', *, *, #15932, .T. ) ;
#23067=CIRCLE ( 'NONE', #46003, 0.1003937007874011050 ) ;
#23129=LINE ( 'NONE', #8737, #20637 ) ;
#23152=LINE ( 'NONE', #11671, #24844 ) ;
#23184=STYLED_ITEM ( 'NONE', ( #14086 ), #3862 ) ;
#23256=DIRECTION ( 'NONE',  ( -3.494233027178531125E-15, -1.000000000000000000, 0.000000000000000000 ) ) ;
#23273=CIRCLE ( 'NONE', #2593, 0.1574803149606291142 ) ;
#23277=ADVANCED_FACE ( 'NONE', ( #7244 ), #25935, .T. ) ;
#23328=EDGE_CURVE ( 'NONE', #39762, #21208, #4789, .T. ) ;
#23346=DIRECTION ( 'NONE',  ( 0.000000000000000000, 1.000000000000000000, 0.000000000000000000 ) ) ;
#23347=DIRECTION ( 'NONE',  ( -3.494233027178531125E-15, -1.000000000000000000, 0.000000000000000000 ) ) ;
#23361=VERTEX_POINT ( 'NONE', #30912 ) ;
#23414=AXIS2_PLACEMENT_3D ( 'NONE', #38166, #26467, #31003 ) ;
#23506=VECTOR ( 'NONE', #47181, 39.37007874015748143 ) ;
#23556=ADVANCED_FACE ( 'NONE', ( #25770 ), #21925, .F. ) ;
#23574=CARTESIAN_POINT ( 'NONE',  ( -0.5555748031496045014, 0.6449983665207589256, -0.06082000038405668829 ) ) ;
#23764=FACE_OUTER_BOUND ( 'NONE', #26108, .T. ) ;
#23806=DIRECTION ( 'NONE',  ( 0.000000000000000000, 0.000000000000000000, 1.000000000000000000 ) ) ;
#23816=VERTEX_POINT ( 'NONE', #3650 ) ;
#23828=CARTESIAN_POINT ( 'NONE',  ( -7.957671378281915615E-17, 0.1574803149606340824, -0.3937007874015748254 ) ) ;
#24006=DIRECTION ( 'NONE',  ( -3.494233027178502331E-15, -1.000000000000000000, -0.000000000000000000 ) ) ;
#24089=CARTESIAN_POINT ( 'NONE',  ( 1.614954907737318939E-16, 0.1574803149606340824, 0.3937007874015748254 ) ) ;
#24139=EDGE_LOOP ( 'NONE', ( #9338, #31343 ) ) ;
#24186=DIRECTION ( 'NONE',  ( 0.000000000000000000, 1.000000000000000000, 0.000000000000000000 ) ) ;
#24206=DIRECTION ( 'NONE',  ( -0.000000000000000000, 1.000000000000000000, -0.000000000000000000 ) ) ;
#24212=FACE_OUTER_BOUND ( 'NONE', #2984, .T. ) ;
#24216=ORIENTED_EDGE ( 'NONE', *, *, #26324, .F. ) ;
#24298=ORIENTED_EDGE ( 'NONE', *, *, #46241, .T. ) ;
#24305=DIRECTION ( 'NONE',  ( 1.000000000000000000, -3.368395098984144529E-15, 0.000000000000000000 ) ) ;
#24573=CARTESIAN_POINT ( 'NONE',  ( -0.3980944881889762477, 0.1574803149606354702, -0.7480314960629921295 ) ) ;
#24630=( NAMED_UNIT ( * ) PLANE_ANGLE_UNIT ( ) SI_UNIT ( $, .RADIAN. ) ) ;
#24779=DIRECTION ( 'NONE',  ( -0.000000000000000000, 1.000000000000000000, -0.000000000000000000 ) ) ;
#24781=ORIENTED_EDGE ( 'NONE', *, *, #37423, .F. ) ;
#24842=DIRECTION ( 'NONE',  ( 1.000000000000000000, 0.000000000000000000, 0.000000000000000000 ) ) ;
#24844=VECTOR ( 'NONE', #26763, 39.37007874015748143 ) ;
#24926=DIRECTION ( 'NONE',  ( 3.469446951953620894E-15, 1.000000000000000000, 0.000000000000000000 ) ) ;
#25041=CARTESIAN_POINT ( 'NONE',  ( -0.3980944881889768028, 5.463695987328542214E-16, -0.7480314960629921295 ) ) ;
#25054=CARTESIAN_POINT ( 'NONE',  ( 0.3980944881889770803, 0.1864803149606326926, -0.7480314960629921295 ) ) ;
#25095=EDGE_CURVE ( 'NONE', #28102, #13381, #11253, .T. ) ;
#25107=EDGE_CURVE ( 'NONE', #33534, #5993, #25637, .T. ) ;
#25265=DIRECTION ( 'NONE',  ( -3.469446951953614189E-15, -1.000000000000000000, 0.000000000000000000 ) ) ;
#25294=VERTEX_POINT ( 'NONE', #1618 ) ;
#25327=ORIENTED_EDGE ( 'NONE', *, *, #31858, .F. ) ;
#25340=CARTESIAN_POINT ( 'NONE',  ( -0.3980944881889745268, 0.6449983665207583705, -0.06082000038405668829 ) ) ;
#25371=ORIENTED_EDGE ( 'NONE', *, *, #18600, .F. ) ;
#25385=DIRECTION ( 'NONE',  ( 0.000000000000000000, 0.000000000000000000, 1.000000000000000000 ) ) ;
#25415=CARTESIAN_POINT ( 'NONE',  ( -0.5555748031496053896, 0.3833307086614213266, 0.7480314960629921295 ) ) ;
#25455=CARTESIAN_POINT ( 'NONE',  ( 0.3980944881889810216, 1.332209862199691841, -0.06082000038405670217 ) ) ;
#25514=EDGE_CURVE ( 'NONE', #4077, #3165, #23273, .T. ) ;
#25524=PRODUCT_DEFINITION_FORMATION_WITH_SPECIFIED_SOURCE ( 'ANY', '', #26085, .NOT_KNOWN. ) ;
#25581=DIRECTION ( 'NONE',  ( -0.000000000000000000, 1.000000000000000000, -0.000000000000000000 ) ) ;
#25637=LINE ( 'NONE', #11730, #15623 ) ;
#25646=DIRECTION ( 'NONE',  ( 1.000000000000000000, -3.469446951953625627E-15, -0.000000000000000000 ) ) ;
#25692=CARTESIAN_POINT ( 'NONE',  ( 0.000000000000000000, 0.000000000000000000, 0.000000000000000000 ) ) ;
#25693=DIRECTION ( 'NONE',  ( 3.469446951953620894E-15, 1.000000000000000000, 0.000000000000000000 ) ) ;
#25770=FACE_OUTER_BOUND ( 'NONE', #43366, .T. ) ;
#25835=ORIENTED_EDGE ( 'NONE', *, *, #40661, .T. ) ;
#25886=VECTOR ( 'NONE', #14458, 39.37007874015748143 ) ;
#25912=AXIS2_PLACEMENT_3D ( 'NONE', #18898, #37344, #18430 ) ;
#25930=CARTESIAN_POINT ( 'NONE',  ( -0.3980944881889741382, 0.7681739484881655589, -0.04983111751016786051 ) ) ;
#25935=PLANE ( 'NONE',  #36931 ) ;
#25963=LINE ( 'NONE', #32705, #27523 ) ;
#25988=EDGE_CURVE ( 'NONE', #21943, #19046, #31997, .T. ) ;
#26025=EDGE_LOOP ( 'NONE', ( #29759, #16409 ) ) ;
#26030=CYLINDRICAL_SURFACE ( 'NONE', #15215, 0.1003937007874011050 ) ;
#26084=DIRECTION ( 'NONE',  ( -3.469446951953590129E-15, -1.000000000000000000, 0.000000000000000000 ) ) ;
#26085=PRODUCT ( 'Hook Bracket', 'Hook Bracket', '', ( #31237 ) ) ;
#26108=EDGE_LOOP ( 'NONE', ( #4561, #38853, #36006, #32379 ) ) ;
#26159=AXIS2_PLACEMENT_3D ( 'NONE', #10257, #43528, #10743 ) ;
#26195=AXIS2_PLACEMENT_3D ( 'NONE', #6407, #21019, #35667 ) ;
#26203=ORIENTED_EDGE ( 'NONE', *, *, #13858, .F. ) ;
#26206=VERTEX_POINT ( 'NONE', #18780 ) ;
#26209=DIRECTION ( 'NONE',  ( 0.000000000000000000, 0.000000000000000000, -1.000000000000000000 ) ) ;
#26245=CARTESIAN_POINT ( 'NONE',  ( 0.5555748031496103856, 0.7681739484881628943, -0.04983111751016747887 ) ) ;
#26246=DIRECTION ( 'NONE',  ( 0.000000000000000000, -0.000000000000000000, 1.000000000000000000 ) ) ;
#26324=EDGE_CURVE ( 'NONE', #19773, #39762, #15687, .T. ) ;
#26346=DIRECTION ( 'NONE',  ( 0.000000000000000000, 0.000000000000000000, -1.000000000000000000 ) ) ;
#26445=ORIENTED_EDGE ( 'NONE', *, *, #1198, .T. ) ;
#26463=AXIS2_PLACEMENT_3D ( 'NONE', #9056, #13371, #38526 ) ;
#26467=DIRECTION ( 'NONE',  ( -1.000000000000000000, 3.469446951953614189E-15, 0.000000000000000000 ) ) ;
#26473=CARTESIAN_POINT ( 'NONE',  ( 0.5555748031496114958, 1.061695335278752150, -0.02376411959061622975 ) ) ;
#26522=AXIS2_PLACEMENT_3D ( 'NONE', #8491, #11639, #44900 ) ;
#26559=ORIENTED_EDGE ( 'NONE', *, *, #18600, .T. ) ;
#26632=CARTESIAN_POINT ( 'NONE',  ( -7.957671378281915615E-17, 0.1574803149606340824, -0.3937007874015748254 ) ) ;
#26697=ADVANCED_FACE ( 'NONE', ( #35485 ), #31895, .T. ) ;
#26730=ORIENTED_EDGE ( 'NONE', *, *, #43153, .F. ) ;
#26756=EDGE_CURVE ( 'NONE', #43268, #10222, #19777, .T. ) ;
#26763=DIRECTION ( 'NONE',  ( -1.267059173938978811E-30, -3.652049423109077687E-16, 1.000000000000000000 ) ) ;
#26788=DIRECTION ( 'NONE',  ( 0.000000000000000000, -0.4344452574044149196, 0.9006982393225888561 ) ) ;
#26855=AXIS2_PLACEMENT_3D ( 'NONE', #23574, #45116, #5832 ) ;
#26875=VECTOR ( 'NONE', #34205, 39.37007874015748143 ) ;
#26968=DIRECTION ( 'NONE',  ( 1.000000000000000000, -3.469446951953626022E-15, -0.000000000000000000 ) ) ;
#27058=VERTEX_POINT ( 'NONE', #34479 ) ;
#27083=CARTESIAN_POINT ( 'NONE',  ( -0.3980944881889753040, 0.4370297686271548687, 0.6367018223237034258 ) ) ;
#27119=CYLINDRICAL_SURFACE ( 'NONE', #13425, 0.1003937007874011050 ) ;
#27174=ORIENTED_EDGE ( 'NONE', *, *, #13429, .F. ) ;
#27200=LINE ( 'NONE', #38426, #13618 ) ;
#27232=CIRCLE ( 'NONE', #41699, 0.1574803149606291142 ) ;
#27264=DIRECTION ( 'NONE',  ( 3.469446951953626022E-15, 1.000000000000000000, 0.000000000000000000 ) ) ;
#27280=VERTEX_POINT ( 'NONE', #17670 ) ;
#27403=ORIENTED_EDGE ( 'NONE', *, *, #40234, .T. ) ;
#27479=DIRECTION ( 'NONE',  ( -1.000000000000000000, 3.469446951953613794E-15, 0.000000000000000000 ) ) ;
#27523=VECTOR ( 'NONE', #21411, 39.37007874015748143 ) ;
#27577=VERTEX_POINT ( 'NONE', #29229 ) ;
#27633=DIRECTION ( 'NONE',  ( 1.000000000000000000, -3.469446951953625627E-15, -0.000000000000000000 ) ) ;
#27683=DIRECTION ( 'NONE',  ( -3.478357113474434231E-15, -1.000000000000000000, 0.000000000000000000 ) ) ;
#27692=AXIS2_PLACEMENT_3D ( 'NONE', #6325, #42031, #20945 ) ;
#27720=VECTOR ( 'NONE', #7309, 39.37007874015748143 ) ;
#27824=CARTESIAN_POINT ( 'NONE',  ( -7.957671378281915615E-17, 0.1574803149606340824, -0.3937007874015748254 ) ) ;
#27840=PLANE ( 'NONE',  #7975 ) ;
#27886=DIRECTION ( 'NONE',  ( 0.000000000000000000, 0.000000000000000000, -1.000000000000000000 ) ) ;
#27928=AXIS2_PLACEMENT_3D ( 'NONE', #12349, #26968, #12593 ) ;
#27998=LINE ( 'NONE', #38982, #28008 ) ;
#28008=VECTOR ( 'NONE', #38051, 39.37007874015748854 ) ;
#28102=VERTEX_POINT ( 'NONE', #11147 ) ;
#28159=FACE_OUTER_BOUND ( 'NONE', #2993, .T. ) ;
#28202=ORIENTED_EDGE ( 'NONE', *, *, #32209, .T. ) ;
#28238=FILL_AREA_STYLE ('',( #6641 ) ) ;
#28281=ORIENTED_EDGE ( 'NONE', *, *, #33690, .T. ) ;
#28375=EDGE_CURVE ( 'NONE', #43268, #36366, #41042, .T. ) ;
#28415=CARTESIAN_POINT ( 'NONE',  ( -6.728203135043436585E-17, 0.1564960629921311464, -0.4940944881889759444 ) ) ;
#28451=ORIENTED_EDGE ( 'NONE', *, *, #25514, .T. ) ;
#28557=ORIENTED_EDGE ( 'NONE', *, *, #25988, .F. ) ;
#28592=LENGTH_MEASURE_WITH_UNIT ( LENGTH_MEASURE( 0.02539999999999999897 ), #29073 ) ;
#28715=ORIENTED_EDGE ( 'NONE', *, *, #12960, .T. ) ;
#28765=LINE ( 'NONE', #39724, #37942 ) ;
#28946=DIRECTION ( 'NONE',  ( 0.000000000000000000, 0.000000000000000000, 1.000000000000000000 ) ) ;
#28951=ORIENTED_EDGE ( 'NONE', *, *, #39324, .T. ) ;
#29029=FACE_OUTER_BOUND ( 'NONE', #11403, .T. ) ;
#29073=( LENGTH_UNIT ( ) NAMED_UNIT ( * ) SI_UNIT ( $, .METRE. ) ) ;
#29075=DIRECTION ( 'NONE',  ( -1.000000000000000000, 3.469446951953626022E-15, 0.000000000000000000 ) ) ;
#29155=DIRECTION ( 'NONE',  ( -1.000000000000000000, 0.000000000000000000, 0.000000000000000000 ) ) ;
#29186=VERTEX_POINT ( 'NONE', #34539 ) ;
#29210=AXIS2_PLACEMENT_3D ( 'NONE', #31784, #13105, #13329 ) ;
#29229=CARTESIAN_POINT ( 'NONE',  ( -0.5555748031496058337, 0.2597269656108975311, 0.7480314960629921295 ) ) ;
#29309=CARTESIAN_POINT ( 'NONE',  ( -6.716149524815622026E-17, 0.1574803149606340824, -0.4950787401574787139 ) ) ;
#29324=ORIENTED_EDGE ( 'NONE', *, *, #2109, .F. ) ;
#29361=CIRCLE ( 'NONE', #9400, 0.1013779527559039162 ) ;
#29381=AXIS2_PLACEMENT_3D ( 'NONE', #10667, #16960, #31830 ) ;
#29507=VECTOR ( 'NONE', #44385, 39.37007874015748143 ) ;
#29669=ORIENTED_EDGE ( 'NONE', *, *, #16196, .T. ) ;
#29714=CARTESIAN_POINT ( 'NONE',  ( -6.728203135043436585E-17, 0.1564960629921311464, -0.4940944881889759444 ) ) ;
#29750=CARTESIAN_POINT ( 'NONE',  ( -0.3690944881889761109, 0.1864803149606354127, -0.06082000038405668829 ) ) ;
#29759=ORIENTED_EDGE ( 'NONE', *, *, #15828, .T. ) ;
#29792=CARTESIAN_POINT ( 'NONE',  ( 0.3690944881889770546, 0.1574803149606328057, -0.7480314960629921295 ) ) ;
#29831=DIRECTION ( 'NONE',  ( 0.000000000000000000, 1.000000000000000000, 0.000000000000000000 ) ) ;
#29908=LINE ( 'NONE', #44686, #4919 ) ;
#29915=CONICAL_SURFACE ( 'NONE', #20701, 0.1003937007874011050, 0.7853981633973787790 ) ;
#29942=CARTESIAN_POINT ( 'NONE',  ( 0.3980944881889773024, 0.2597269656108940894, 0.5511811023622046335 ) ) ;
#29964=CARTESIAN_POINT ( 'NONE',  ( 0.3690944881889770546, 0.1574803149606328057, -0.7480314960629921295 ) ) ;
#29972=ORIENTED_EDGE ( 'NONE', *, *, #10960, .F. ) ;
#30080=DIRECTION ( 'NONE',  ( 1.000000000000000000, -3.368395098984144529E-15, 0.000000000000000000 ) ) ;
#30299=EDGE_CURVE ( 'NONE', #26206, #23816, #39025, .T. ) ;
#30301=DIRECTION ( 'NONE',  ( 0.000000000000000000, 0.000000000000000000, 1.000000000000000000 ) ) ;
#30373=CARTESIAN_POINT ( 'NONE',  ( 0.5555748031496086092, 0.2597269656108935343, 0.7480314960629921295 ) ) ;
#30426=AXIS2_PLACEMENT_3D ( 'NONE', #29750, #44298, #19387 ) ;
#30429=DIRECTION ( 'NONE',  ( 1.000000000000000000, -3.469446951953614189E-15, -0.000000000000000000 ) ) ;
#30436=ADVANCED_FACE ( 'NONE', ( #15527 ), #22451, .T. ) ;
#30455=VERTEX_POINT ( 'NONE', #41345 ) ;
#30656=EDGE_CURVE ( 'NONE', #9464, #11301, #31100, .T. ) ;
#30707=FACE_OUTER_BOUND ( 'NONE', #17451, .T. ) ;
#30767=EDGE_LOOP ( 'NONE', ( #2886, #29669, #5466, #43721, #28202, #32234, #22996, #12117 ) ) ;
#30801=CARTESIAN_POINT ( 'NONE',  ( 1.614954907737318939E-16, 0.1564960629921311464, 0.3937007874015748254 ) ) ;
#30818=DIRECTION ( 'NONE',  ( 3.385139170096243171E-15, 1.000000000000000000, -0.000000000000000000 ) ) ;
#30855=CARTESIAN_POINT ( 'NONE',  ( -0.5555748031496045014, 0.6449983665207589256, -0.7480314960629921295 ) ) ;
#30865=DIRECTION ( 'NONE',  ( 1.000000000000000000, -3.469446951953613794E-15, -0.000000000000000000 ) ) ;
#30912=CARTESIAN_POINT ( 'NONE',  ( -7.957671378281915615E-17, 0.1564960629921311464, -0.2933070866141737065 ) ) ;
#31003=DIRECTION ( 'NONE',  ( -3.478357113474434231E-15, -1.000000000000000000, 0.000000000000000000 ) ) ;
#31041=LINE ( 'NONE', #45382, #45607 ) ;
#31100=LINE ( 'NONE', #34221, #42052 ) ;
#31148=ORIENTED_EDGE ( 'NONE', *, *, #46241, .F. ) ;
#31237=PRODUCT_CONTEXT ( 'NONE', #8584, 'mechanical' ) ;
#31285=DIRECTION ( 'NONE',  ( 0.000000000000000000, 0.000000000000000000, 1.000000000000000000 ) ) ;
#31288=ORIENTED_EDGE ( 'NONE', *, *, #31492, .F. ) ;
#31336=CARTESIAN_POINT ( 'NONE',  ( 0.5555748031496086092, 0.2597269656108935343, 0.5511811023622046335 ) ) ;
#31343=ORIENTED_EDGE ( 'NONE', *, *, #45389, .T. ) ;
#31484=FACE_OUTER_BOUND ( 'NONE', #44322, .T. ) ;
#31492=EDGE_CURVE ( 'NONE', #22330, #33536, #44122, .T. ) ;
#31515=ORIENTED_EDGE ( 'NONE', *, *, #9639, .T. ) ;
#31531=DIRECTION ( 'NONE',  ( 1.000000000000000000, 0.000000000000000000, 0.000000000000000000 ) ) ;
#31557=FACE_OUTER_BOUND ( 'NONE', #44081, .T. ) ;
#31568=DIRECTION ( 'NONE',  ( 0.000000000000000000, -0.000000000000000000, 1.000000000000000000 ) ) ;
#31579=CARTESIAN_POINT ( 'NONE',  ( 0.5555748031496086092, 0.2597269656108935343, 0.7480314960629921295 ) ) ;
#31601=( GEOMETRIC_REPRESENTATION_CONTEXT ( 3 ) GLOBAL_UNCERTAINTY_ASSIGNED_CONTEXT ( ( #44658 ) ) GLOBAL_UNIT_ASSIGNED_CONTEXT ( ( #39792, #6742, #17773 ) ) REPRESENTATION_CONTEXT ( 'NONE', 'WORKASPACE' ) ) ;
#31602=CARTESIAN_POINT ( 'NONE',  ( 0.3690944881889778317, 3.409318977613033647E-15, -0.7480314960629921295 ) ) ;
#31654=CARTESIAN_POINT ( 'NONE',  ( 0.5555748031496077211, 2.762335417273526192E-15, -0.7480314960629921295 ) ) ;
#31678=CARTESIAN_POINT ( 'NONE',  ( -7.957671378281915615E-17, 0.1564960629921311464, -0.2933070866141737065 ) ) ;
#31753=EDGE_LOOP ( 'NONE', ( #15969, #509, #6647, #43304 ) ) ;
#31769=ORIENTED_EDGE ( 'NONE', *, *, #39100, .T. ) ;
#31784=CARTESIAN_POINT ( 'NONE',  ( 0.3980944881889805775, 1.194414586609139795, -0.06082000038405787484 ) ) ;
#31787=LINE ( 'NONE', #14027, #15450 ) ;
#31830=DIRECTION ( 'NONE',  ( -3.478357113474434231E-15, -1.000000000000000000, 0.000000000000000000 ) ) ;
#31831=AXIS2_PLACEMENT_3D ( 'NONE', #2608, #46455, #3075 ) ;
#31858=EDGE_CURVE ( 'NONE', #36803, #27280, #15989, .T. ) ;
#31883=ORIENTED_EDGE ( 'NONE', *, *, #1809, .T. ) ;
#31895=CYLINDRICAL_SURFACE ( 'NONE', #35562, 0.6872114956789353579 ) ;
#31956=VERTEX_POINT ( 'NONE', #11916 ) ;
#31992=EDGE_CURVE ( 'NONE', #36366, #1004, #45418, .T. ) ;
#31997=LINE ( 'NONE', #20950, #7999 ) ;
#32082=VECTOR ( 'NONE', #16939, 39.37007874015748854 ) ;
#32110=ADVANCED_FACE ( 'NONE', ( #5405, #38245, #20027 ), #35372, .F. ) ;
#32209=EDGE_CURVE ( 'NONE', #33762, #46575, #15374, .T. ) ;
#32229=DIRECTION ( 'NONE',  ( 0.000000000000000000, 0.000000000000000000, 1.000000000000000000 ) ) ;
#32234=ORIENTED_EDGE ( 'NONE', *, *, #35872, .T. ) ;
#32379=ORIENTED_EDGE ( 'NONE', *, *, #19218, .T. ) ;
#32542=EDGE_CURVE ( 'NONE', #40321, #21943, #38296, .T. ) ;
#32578=ORIENTED_EDGE ( 'NONE', *, *, #44779, .F. ) ;
#32591=CARTESIAN_POINT ( 'NONE',  ( -0.3690944881889767215, 5.970426471673286898E-15, -0.7480314960629921295 ) ) ;
#32652=DIRECTION ( 'NONE',  ( 0.000000000000000000, 0.000000000000000000, 1.000000000000000000 ) ) ;
#32705=CARTESIAN_POINT ( 'NONE',  ( 0.3980944881889764142, 2.762335417273529347E-15, 0.7480314960629921295 ) ) ;
#32728=CARTESIAN_POINT ( 'NONE',  ( 0.3690944881889778317, 3.409318977613033647E-15, -0.7480314960629921295 ) ) ;
#32739=ORIENTED_EDGE ( 'NONE', *, *, #44779, .T. ) ;
#32966=DIRECTION ( 'NONE',  ( -3.124924761047754241E-15, -0.9006982393225890782, -0.4344452574044144755 ) ) ;
#32997=EDGE_CURVE ( 'NONE', #3165, #33762, #41264, .T. ) ;
#33053=DIRECTION ( 'NONE',  ( 3.469446951953614189E-15, 1.000000000000000000, 1.040834085586084257E-15 ) ) ;
#33090=DIRECTION ( 'NONE',  ( 0.000000000000000000, 1.000000000000000000, 0.000000000000000000 ) ) ;
#33100=ORIENTED_EDGE ( 'NONE', *, *, #31858, .T. ) ;
#33220=ORIENTED_EDGE ( 'NONE', *, *, #25514, .F. ) ;
#33245=ORIENTED_EDGE ( 'NONE', *, *, #25107, .T. ) ;
#33359=CIRCLE ( 'NONE', #26463, 0.6872114956789353579 ) ;
#33425=LINE ( 'NONE', #538, #29507 ) ;
#33469=EDGE_LOOP ( 'NONE', ( #18106, #24298 ) ) ;
#33484=CARTESIAN_POINT ( 'NONE',  ( 0.5555748031496099415, 0.6449983665207552619, -0.7480314960629921295 ) ) ;
#33510=DIRECTION ( 'NONE',  ( -1.000000000000000000, 0.000000000000000000, 0.000000000000000000 ) ) ;
#33534=VERTEX_POINT ( 'NONE', #8408 ) ;
#33536=VERTEX_POINT ( 'NONE', #37651 ) ;
#33641=EDGE_LOOP ( 'NONE', ( #43368, #6251, #20039, #46342 ) ) ;
#33690=EDGE_CURVE ( 'NONE', #27577, #7744, #42224, .T. ) ;
#33762=VERTEX_POINT ( 'NONE', #14092 ) ;
#33940=VERTEX_POINT ( 'NONE', #397 ) ;
#33958=PLANE ( 'NONE',  #14776 ) ;
#33977=VERTEX_POINT ( 'NONE', #18899 ) ;
#34066=AXIS2_PLACEMENT_3D ( 'NONE', #30801, #33090, #39526 ) ;
#34112=CARTESIAN_POINT ( 'NONE',  ( 1.614954907737318939E-16, 0.1564960629921311464, 0.3937007874015748254 ) ) ;
#34181=LINE ( 'NONE', #41787, #19852 ) ;
#34205=DIRECTION ( 'NONE',  ( 1.000000000000000000, -3.469446951953625233E-15, -0.000000000000000000 ) ) ;
#34221=CARTESIAN_POINT ( 'NONE',  ( -0.3980944881889762477, 0.1574803149606354702, 0.7480314960629921295 ) ) ;
#34275=EDGE_LOOP ( 'NONE', ( #10301, #33245, #42749, #14596 ) ) ;
#34374=LINE ( 'NONE', #26245, #42638 ) ;
#34433=LINE ( 'NONE', #19571, #3778 ) ;
#34479=CARTESIAN_POINT ( 'NONE',  ( 0.3980944881889773024, 0.2597269656108940894, 0.7480314960629921295 ) ) ;
#34539=CARTESIAN_POINT ( 'NONE',  ( -0.5555748031496061667, 0.1864803149606359678, 0.7480314960629921295 ) ) ;
#34567=VECTOR ( 'NONE', #37235, 39.37007874015748143 ) ;
#34571=VERTEX_POINT ( 'NONE', #25054 ) ;
#34605=CARTESIAN_POINT ( 'NONE',  ( 1.614954907737318939E-16, 0.1564960629921311464, 0.3937007874015748254 ) ) ;
#34728=EDGE_LOOP ( 'NONE', ( #16476, #8510 ) ) ;
#34801=LINE ( 'NONE', #31678, #9915 ) ;
#34983=ORIENTED_EDGE ( 'NONE', *, *, #44187, .T. ) ;
#35023=ADVANCED_FACE ( 'NONE', ( #9692 ), #17339, .T. ) ;
#35035=CARTESIAN_POINT ( 'NONE',  ( -0.3980944881889731390, 1.061695335278756147, -0.02376411959061705201 ) ) ;
#35038=ORIENTED_EDGE ( 'NONE', *, *, #45869, .T. ) ;
#35096=DIRECTION ( 'NONE',  ( 1.267059173938974432E-30, 3.652049423109077687E-16, -1.000000000000000000 ) ) ;
#35111=CARTESIAN_POINT ( 'NONE',  ( -7.957671378281915615E-17, 0.1564960629921311464, -0.3937007874015748254 ) ) ;
#35145=PLANE ( 'NONE',  #6188 ) ;
#35155=DIRECTION ( 'NONE',  ( -1.267059173938974432E-30, -3.652049423109077687E-16, 1.000000000000000000 ) ) ;
#35170=DIRECTION ( 'NONE',  ( 0.000000000000000000, -0.000000000000000000, 1.000000000000000000 ) ) ;
#35195=SURFACE_SIDE_STYLE ('',( #9554 ) ) ;
#35199=CARTESIAN_POINT ( 'NONE',  ( -0.3980944881889736386, 0.9100161909011718064, 0.01858545845903165558 ) ) ;
#35238=PLANE ( 'NONE',  #31831 ) ;
#35334=DIRECTION ( 'NONE',  ( -3.469446951953614189E-15, -1.000000000000000000, 0.000000000000000000 ) ) ;
#35337=CIRCLE ( 'NONE', #26159, 0.1864803149606298893 ) ;
#35372=PLANE ( 'NONE',  #4633 ) ;
#35389=ORIENTED_EDGE ( 'NONE', *, *, #23328, .F. ) ;
#35426=ORIENTED_EDGE ( 'NONE', *, *, #21966, .T. ) ;
#35485=FACE_OUTER_BOUND ( 'NONE', #119, .T. ) ;
#35496=VERTEX_POINT ( 'NONE', #42186 ) ;
#35510=ADVANCED_FACE ( 'NONE', ( #23764 ), #37426, .F. ) ;
#35520=ORIENTED_EDGE ( 'NONE', *, *, #44180, .T. ) ;
#35562=AXIS2_PLACEMENT_3D ( 'NONE', #44525, #25646, #40687 ) ;
#35587=AXIS2_PLACEMENT_3D ( 'NONE', #7158, #37319, #26084 ) ;
#35607=LINE ( 'NONE', #25041, #27720 ) ;
#35657=AXIS2_PLACEMENT_3D ( 'NONE', #25340, #46642, #44392 ) ;
#35667=DIRECTION ( 'NONE',  ( -3.469446951953631938E-15, -1.000000000000000000, 0.000000000000000000 ) ) ;
#35716=LINE ( 'NONE', #25415, #8676 ) ;
#35721=ORIENTED_EDGE ( 'NONE', *, *, #46571, .T. ) ;
#35756=LINE ( 'NONE', #2896, #47106 ) ;
#35805=CARTESIAN_POINT ( 'NONE',  ( -7.957671378281915615E-17, -8.878505979408855953E-16, -0.3937007874015748254 ) ) ;
#35872=EDGE_CURVE ( 'NONE', #46575, #30455, #46129, .T. ) ;
#36006=ORIENTED_EDGE ( 'NONE', *, *, #254, .F. ) ;
#36018=ORIENTED_EDGE ( 'NONE', *, *, #42928, .T. ) ;
#36096=VECTOR ( 'NONE', #41035, 39.37007874015748143 ) ;
#36176=ORIENTED_EDGE ( 'NONE', *, *, #9551, .F. ) ;
#36366=VERTEX_POINT ( 'NONE', #42681 ) ;
#36406=DIRECTION ( 'NONE',  ( -1.000000000000000000, 3.469446951953626022E-15, 0.000000000000000000 ) ) ;
#36439=CARTESIAN_POINT ( 'NONE',  ( 1.614954907737318939E-16, -8.878505979408855953E-16, 0.3937007874015748254 ) ) ;
#36513=ORIENTED_EDGE ( 'NONE', *, *, #6936, .F. ) ;
#36803=VERTEX_POINT ( 'NONE', #5990 ) ;
#36898=ORIENTED_EDGE ( 'NONE', *, *, #26324, .T. ) ;
#36931=AXIS2_PLACEMENT_3D ( 'NONE', #498, #15391, #18494 ) ;
#36932=ORIENTED_EDGE ( 'NONE', *, *, #42928, .F. ) ;
#37080=VECTOR ( 'NONE', #37469, 39.37007874015748854 ) ;
#37152=DIRECTION ( 'NONE',  ( -0.000000000000000000, 1.000000000000000000, -0.000000000000000000 ) ) ;
#37169=EDGE_CURVE ( 'NONE', #29186, #27577, #35716, .T. ) ;
#37235=DIRECTION ( 'NONE',  ( 1.000000000000000000, -3.469446951953625233E-15, -0.000000000000000000 ) ) ;
#37319=DIRECTION ( 'NONE',  ( -1.000000000000000000, 3.469446951953614189E-15, 0.000000000000000000 ) ) ;
#37344=DIRECTION ( 'NONE',  ( -0.000000000000000000, 1.000000000000000000, -0.000000000000000000 ) ) ;
#37391=ORIENTED_EDGE ( 'NONE', *, *, #14169, .F. ) ;
#37423=EDGE_CURVE ( 'NONE', #23816, #9464, #22740, .T. ) ;
#37426=CYLINDRICAL_SURFACE ( 'NONE', #14757, 0.1574803149606301966 ) ;
#37469=DIRECTION ( 'NONE',  ( 1.541976423090495042E-15, 0.4344452574044144755, -0.9006982393225890782 ) ) ;
#37501=ADVANCED_FACE ( 'NONE', ( #5350 ), #45838, .T. ) ;
#37598=ORIENTED_EDGE ( 'NONE', *, *, #7618, .F. ) ;
#37651=CARTESIAN_POINT ( 'NONE',  ( -0.3980944881889721398, 1.332209862199693839, -0.06082000038405668829 ) ) ;
#37706=ADVANCED_FACE ( 'NONE', ( #1514 ), #10337, .F. ) ;
#37835=EDGE_CURVE ( 'NONE', #10222, #43268, #12673, .T. ) ;
#37865=CARTESIAN_POINT ( 'NONE',  ( -0.5555748031496052786, 0.4370297686271554238, 0.6367018223237034258 ) ) ;
#37942=VECTOR ( 'NONE', #6910, 39.37007874015748143 ) ;
#37956=PLANE ( 'NONE',  #26855 ) ;
#37973=CIRCLE ( 'NONE', #26522, 0.1968503937007874405 ) ;
#37982=ORIENTED_EDGE ( 'NONE', *, *, #39324, .F. ) ;
#38051=DIRECTION ( 'NONE',  ( 1.541976423090495042E-15, 0.4344452574044150306, -0.9006982393225888561 ) ) ;
#38159=ORIENTED_EDGE ( 'NONE', *, *, #12960, .F. ) ;
#38166=CARTESIAN_POINT ( 'NONE',  ( 0.5555748031496099415, 0.6449983665207552619, -0.06082000038405668829 ) ) ;
#38168=VECTOR ( 'NONE', #789, 39.37007874015748143 ) ;
#38210=EDGE_CURVE ( 'NONE', #5993, #23361, #6558, .T. ) ;
#38245=FACE_BOUND ( 'NONE', #33469, .T. ) ;
#38264=APPLICATION_CONTEXT ( 'automotive_design' ) ;
#38296=LINE ( 'NONE', #31602, #39121 ) ;
#38379=ORIENTED_EDGE ( 'NONE', *, *, #6936, .T. ) ;
#38426=CARTESIAN_POINT ( 'NONE',  ( 0.5555748031496099415, 0.6449983665207552619, -0.7480314960629921295 ) ) ;
#38455=DIRECTION ( 'NONE',  ( 0.000000000000000000, 1.000000000000000000, 0.000000000000000000 ) ) ;
#38464=CARTESIAN_POINT ( 'NONE',  ( 0.3690944881889771101, 0.1864803149606328037, -0.7480314960629921295 ) ) ;
#38526=DIRECTION ( 'NONE',  ( 3.478357113474434231E-15, 1.000000000000000000, 0.000000000000000000 ) ) ;
#38556=CARTESIAN_POINT ( 'NONE',  ( 1.737901732061166719E-16, -8.878505979408855953E-16, 0.2933070866141737065 ) ) ;
#38629=ORIENTED_EDGE ( 'NONE', *, *, #44244, .T. ) ;
#38695=ORIENTED_EDGE ( 'NONE', *, *, #686, .F. ) ;
#38698=CARTESIAN_POINT ( 'NONE',  ( 0.3980944881889790787, 0.7681739484881634494, -0.04983111751016747887 ) ) ;
#38707=LINE ( 'NONE', #13531, #41394 ) ;
#38733=CARTESIAN_POINT ( 'NONE',  ( 0.3980944881889770248, 0.1864803149606327204, 0.7480314960629921295 ) ) ;
#38737=ADVANCED_BREP_SHAPE_REPRESENTATION ( 'Hook Bracket', ( #3862, #20860 ), #31601 ) ;
#38748=ORIENTED_EDGE ( 'NONE', *, *, #7618, .T. ) ;
#38780=DIRECTION ( 'NONE',  ( -3.469446951953608272E-15, -1.000000000000000000, 0.000000000000000000 ) ) ;
#38848=VERTEX_POINT ( 'NONE', #38733 ) ;
#38849=ORIENTED_EDGE ( 'NONE', *, *, #32209, .F. ) ;
#38853=ORIENTED_EDGE ( 'NONE', *, *, #44187, .F. ) ;
#38982=CARTESIAN_POINT ( 'NONE',  ( 0.5555748031496089423, 0.3833307086614172743, 0.7480314960629921295 ) ) ;
#39007=CIRCLE ( 'NONE', #6852, 0.02900000000000001882 ) ;
#39025=CIRCLE ( 'NONE', #19903, 0.02900000000000001882 ) ;
#39035=EDGE_CURVE ( 'NONE', #9464, #33977, #449, .T. ) ;
#39100=EDGE_CURVE ( 'NONE', #19773, #31956, #37973, .T. ) ;
#39121=VECTOR ( 'NONE', #16731, 39.37007874015748143 ) ;
#39124=ORIENTED_EDGE ( 'NONE', *, *, #37169, .T. ) ;
#39229=CARTESIAN_POINT ( 'NONE',  ( 0.5555748031496091643, 0.4370297686271512605, 0.6367018223237037589 ) ) ;
#39319=EDGE_LOOP ( 'NONE', ( #44502, #45871, #31515, #9280 ) ) ;
#39322=VERTEX_POINT ( 'NONE', #8731 ) ;
#39324=EDGE_CURVE ( 'NONE', #28102, #39322, #31041, .T. ) ;
#39377=DIRECTION ( 'NONE',  ( 0.000000000000000000, 0.000000000000000000, 1.000000000000000000 ) ) ;
#39466=LENGTH_MEASURE_WITH_UNIT ( LENGTH_MEASURE( 0.02539999999999999897 ), #17431 ) ;
#39475=VERTEX_POINT ( 'NONE', #29792 ) ;
#39490=AXIS2_PLACEMENT_3D ( 'NONE', #6355, #17865, #10696 ) ;
#39500=DIRECTION ( 'NONE',  ( 3.469446951953631938E-15, 1.000000000000000000, 0.000000000000000000 ) ) ;
#39526=DIRECTION ( 'NONE',  ( 0.000000000000000000, 0.000000000000000000, 1.000000000000000000 ) ) ;
#39603=DIRECTION ( 'NONE',  ( -1.000000000000000000, 3.469446951953625627E-15, 0.000000000000000000 ) ) ;
#39724=CARTESIAN_POINT ( 'NONE',  ( -0.5555748031496030581, 1.061695335278756813, -0.02376411959061705201 ) ) ;
#39762=VERTEX_POINT ( 'NONE', #25930 ) ;
#39771=CIRCLE ( 'NONE', #11520, 0.1013779527559039162 ) ;
#39792=( CONVERSION_BASED_UNIT ( 'INCH', #28592 ) LENGTH_UNIT ( ) NAMED_UNIT ( #1983 ) ) ;
#39811=ORIENTED_EDGE ( 'NONE', *, *, #254, .T. ) ;
#39879=DIRECTION ( 'NONE',  ( 0.000000000000000000, 0.000000000000000000, -1.000000000000000000 ) ) ;
#39908=FACE_OUTER_BOUND ( 'NONE', #34275, .T. ) ;
#39916=AXIS2_PLACEMENT_3D ( 'NONE', #43391, #29075, #25693 ) ;
#39941=DIRECTION ( 'NONE',  ( -1.000000000000000000, 3.469446951953626022E-15, 0.000000000000000000 ) ) ;
#39973=EDGE_CURVE ( 'NONE', #38848, #11301, #19813, .T. ) ;
#40003=VERTEX_POINT ( 'NONE', #39229 ) ;
#40106=AXIS2_PLACEMENT_3D ( 'NONE', #17320, #21627, #3413 ) ;
#40108=DIRECTION ( 'NONE',  ( 0.000000000000000000, 1.000000000000000000, 0.000000000000000000 ) ) ;
#40228=DIRECTION ( 'NONE',  ( 0.000000000000000000, 0.000000000000000000, 1.000000000000000000 ) ) ;
#40234=EDGE_CURVE ( 'NONE', #36366, #35496, #9807, .T. ) ;
#40284=EDGE_CURVE ( 'NONE', #39322, #40321, #16775, .T. ) ;
#40321=VERTEX_POINT ( 'NONE', #32728 ) ;
#40325=AXIS2_PLACEMENT_3D ( 'NONE', #45083, #8924, #30301 ) ;
#40340=CARTESIAN_POINT ( 'NONE',  ( -0.5555748031496040573, 0.7681739484881665581, -0.04983111751016756213 ) ) ;
#40655=DIRECTION ( 'NONE',  ( -0.000000000000000000, 1.000000000000000000, -0.000000000000000000 ) ) ;
#40661=EDGE_CURVE ( 'NONE', #157, #39322, #27200, .T. ) ;
#40687=DIRECTION ( 'NONE',  ( 3.478357113474434231E-15, 1.000000000000000000, 0.000000000000000000 ) ) ;
#40806=DIRECTION ( 'NONE',  ( 0.000000000000000000, 0.4344452574044144755, -0.9006982393225890782 ) ) ;
#40875=EDGE_CURVE ( 'NONE', #7744, #19773, #2457, .T. ) ;
#40924=EDGE_CURVE ( 'NONE', #23361, #5993, #17951, .T. ) ;
#41035=DIRECTION ( 'NONE',  ( -1.000000000000000000, 3.469446951953613794E-15, 0.000000000000000000 ) ) ;
#41039=ORIENTED_EDGE ( 'NONE', *, *, #17399, .F. ) ;
#41042=LINE ( 'NONE', #12811, #38168 ) ;
#41184=DIRECTION ( 'NONE',  ( 0.000000000000000000, 0.000000000000000000, 1.000000000000000000 ) ) ;
#41186=EDGE_CURVE ( 'NONE', #9479, #40003, #29908, .T. ) ;
#41233=EDGE_CURVE ( 'NONE', #33940, #29186, #23152, .T. ) ;
#41264=LINE ( 'NONE', #26473, #36096 ) ;
#41345=CARTESIAN_POINT ( 'NONE',  ( 0.3980944881889786346, 0.6449983665207559280, -0.7480314960629920185 ) ) ;
#41394=VECTOR ( 'NONE', #27479, 39.37007874015748143 ) ;
#41424=DIRECTION ( 'NONE',  ( 1.267059173938978811E-30, 3.652049423109077687E-16, -1.000000000000000000 ) ) ;
#41539=LINE ( 'NONE', #42019, #10002 ) ;
#41669=ORIENTED_EDGE ( 'NONE', *, *, #28375, .T. ) ;
#41699=AXIS2_PLACEMENT_3D ( 'NONE', #43090, #22230, #39500 ) ;
#41711=CARTESIAN_POINT ( 'NONE',  ( -0.5555748031496030581, 1.061695335278756813, -0.02376411959061705201 ) ) ;
#41723=ORIENTED_EDGE ( 'NONE', *, *, #686, .T. ) ;
#41737=SHAPE_DEFINITION_REPRESENTATION ( #14999, #11151 ) ;
#41787=CARTESIAN_POINT ( 'NONE',  ( 0.5555748031496077211, 2.762335417273526192E-15, -0.7480314960629921295 ) ) ;
#41823=AXIS2_PLACEMENT_3D ( 'NONE', #34112, #29831, #26209 ) ;
#42019=CARTESIAN_POINT ( 'NONE',  ( 0.3980944881889776910, 0.3833307086614178294, 0.7480314960629921295 ) ) ;
#42031=DIRECTION ( 'NONE',  ( 1.000000000000000000, -3.469446951953613794E-15, -0.000000000000000000 ) ) ;
#42052=VECTOR ( 'NONE', #1348, 39.37007874015748143 ) ;
#42068=FACE_OUTER_BOUND ( 'NONE', #44330, .T. ) ;
#42186=CARTESIAN_POINT ( 'NONE',  ( 1.737901732061166719E-16, 0.1564960629921311464, 0.2933070866141737065 ) ) ;
#42224=CIRCLE ( 'NONE', #20044, 0.1968503937007874405 ) ;
#42251=ORIENTED_EDGE ( 'NONE', *, *, #4975, .T. ) ;
#42301=AXIS2_PLACEMENT_3D ( 'NONE', #13743, #39603, #35334 ) ;
#42384=DIRECTION ( 'NONE',  ( 1.000000000000000000, -3.368395098984144529E-15, 0.000000000000000000 ) ) ;
#42447=DIRECTION ( 'NONE',  ( -1.000000000000000000, 0.000000000000000000, 0.000000000000000000 ) ) ;
#42499=CARTESIAN_POINT ( 'NONE',  ( 0.5555748031496118289, 1.194414586609139128, -0.06082000038405787484 ) ) ;
#42501=ORIENTED_EDGE ( 'NONE', *, *, #40924, .T. ) ;
#42638=VECTOR ( 'NONE', #11858, 39.37007874015748143 ) ;
#42681=CARTESIAN_POINT ( 'NONE',  ( 1.614954907737318939E-16, 0.1564960629921311464, 0.4940944881889759444 ) ) ;
#42749=ORIENTED_EDGE ( 'NONE', *, *, #38210, .T. ) ;
#42762=CARTESIAN_POINT ( 'NONE',  ( 0.3690944881889784424, 0.1864803149606333310, -0.7480314960629921295 ) ) ;
#42840=CARTESIAN_POINT ( 'NONE',  ( 0.3690944881889784424, 0.1864803149606327759, 0.7480314960629921295 ) ) ;
#42864=DIRECTION ( 'NONE',  ( -1.000000000000000000, 3.469446951953614189E-15, 0.000000000000000000 ) ) ;
#42903=ORIENTED_EDGE ( 'NONE', *, *, #31992, .F. ) ;
#42928=EDGE_CURVE ( 'NONE', #11388, #46575, #35756, .T. ) ;
#42963=CYLINDRICAL_SURFACE ( 'NONE', #5307, 0.1003937007874011050 ) ;
#42986=DIRECTION ( 'NONE',  ( -0.000000000000000000, 0.000000000000000000, -1.000000000000000000 ) ) ;
#43090=CARTESIAN_POINT ( 'NONE',  ( 0.3980944881889795228, 0.9100161909011693639, 0.01858545845903165558 ) ) ;
#43106=EDGE_CURVE ( 'NONE', #40003, #4077, #27998, .T. ) ;
#43109=DIRECTION ( 'NONE',  ( 1.000000000000000000, -3.469446951953625627E-15, -0.000000000000000000 ) ) ;
#43153=EDGE_CURVE ( 'NONE', #22330, #36803, #33359, .T. ) ;
#43262=EDGE_LOOP ( 'NONE', ( #7566, #7621, #5632, #42903 ) ) ;
#43268=VERTEX_POINT ( 'NONE', #13585 ) ;
#43285=CARTESIAN_POINT ( 'NONE',  ( -7.957671378281915615E-17, -8.878505979408855953E-16, -0.3937007874015748254 ) ) ;
#43304=ORIENTED_EDGE ( 'NONE', *, *, #4975, .F. ) ;
#43366=EDGE_LOOP ( 'NONE', ( #11195, #1160, #36898, #45082 ) ) ;
#43368=ORIENTED_EDGE ( 'NONE', *, *, #38210, .F. ) ;
#43378=EDGE_CURVE ( 'NONE', #33536, #27280, #5816, .T. ) ;
#43391=CARTESIAN_POINT ( 'NONE',  ( -0.3980944881889726394, 1.194414586609142237, -0.06082000038405787484 ) ) ;
#43453=CYLINDRICAL_SURFACE ( 'NONE', #326, 0.1968503937007874127 ) ;
#43528=DIRECTION ( 'NONE',  ( -0.000000000000000000, 0.000000000000000000, -1.000000000000000000 ) ) ;
#43547=AXIS2_PLACEMENT_3D ( 'NONE', #42499, #9937, #2719 ) ;
#43590=EDGE_CURVE ( 'NONE', #11388, #157, #17274, .T. ) ;
#43721=ORIENTED_EDGE ( 'NONE', *, *, #9100, .T. ) ;
#43894=ORIENTED_EDGE ( 'NONE', *, *, #43153, .T. ) ;
#43909=LINE ( 'NONE', #18046, #25886 ) ;
#43915=ORIENTED_EDGE ( 'NONE', *, *, #41233, .F. ) ;
#43960=EDGE_LOOP ( 'NONE', ( #39124, #28281, #17468, #39811, #28715, #43894, #18823, #44305 ) ) ;
#44081=EDGE_LOOP ( 'NONE', ( #24216, #31769, #29324, #8483, #1755, #11352, #44903, #35389 ) ) ;
#44122=LINE ( 'NONE', #8355, #11538 ) ;
#44174=ADVANCED_FACE ( 'NONE', ( #24212 ), #35238, .T. ) ;
#44180=EDGE_CURVE ( 'NONE', #21943, #28102, #45567, .T. ) ;
#44187=EDGE_CURVE ( 'NONE', #21109, #21208, #28765, .T. ) ;
#44218=DIRECTION ( 'NONE',  ( -1.000000000000000000, 3.469446951953613794E-15, 0.000000000000000000 ) ) ;
#44244=EDGE_CURVE ( 'NONE', #3165, #11388, #18839, .T. ) ;
#44263=CARTESIAN_POINT ( 'NONE',  ( -0.5555748031496026140, 1.194414586609142903, -0.06082000038405787484 ) ) ;
#44298=DIRECTION ( 'NONE',  ( 0.000000000000000000, 0.000000000000000000, -1.000000000000000000 ) ) ;
#44305=ORIENTED_EDGE ( 'NONE', *, *, #41233, .T. ) ;
#44322=EDGE_LOOP ( 'NONE', ( #27174, #16406, #9738, #31148 ) ) ;
#44330=EDGE_LOOP ( 'NONE', ( #21537, #37982, #13183, #2130 ) ) ;
#44385=DIRECTION ( 'NONE',  ( -1.000000000000000000, 3.469446951953625233E-15, 0.000000000000000000 ) ) ;
#44392=DIRECTION ( 'NONE',  ( 3.478357113474434231E-15, 1.000000000000000000, 0.000000000000000000 ) ) ;
#44441=ORIENTED_EDGE ( 'NONE', *, *, #37169, .F. ) ;
#44502=ORIENTED_EDGE ( 'NONE', *, *, #37835, .F. ) ;
#44525=CARTESIAN_POINT ( 'NONE',  ( -0.5555748031496045014, 0.6449983665207589256, -0.06082000038405668829 ) ) ;
#44579=AXIS2_PLACEMENT_3D ( 'NONE', #40340, #32966, #40806 ) ;
#44590=ORIENTED_EDGE ( 'NONE', *, *, #16350, .F. ) ;
#44635=CARTESIAN_POINT ( 'NONE',  ( -0.5555748031496040573, 0.7681739484881661140, -0.04983111751016786051 ) ) ;
#44658=UNCERTAINTY_MEASURE_WITH_UNIT (LENGTH_MEASURE( 1.000000000000000082E-05 ), #39792, 'distance_accuracy_value', 'NONE') ;
#44686=CARTESIAN_POINT ( 'NONE',  ( 0.5555748031496091643, 0.4370297686271511495, 0.6367018223237037589 ) ) ;
#44779=EDGE_CURVE ( 'NONE', #29186, #19046, #12678, .T. ) ;
#44861=DIRECTION ( 'NONE',  ( -3.469446951953613794E-15, -1.000000000000000000, 0.000000000000000000 ) ) ;
#44900=DIRECTION ( 'NONE',  ( 3.469446951953613794E-15, 1.000000000000000000, 0.000000000000000000 ) ) ;
#44903=ORIENTED_EDGE ( 'NONE', *, *, #46571, .F. ) ;
#44937=DIRECTION ( 'NONE',  ( 0.000000000000000000, 0.7071067811865965336, 0.7071067811864983899 ) ) ;
#44952=DIRECTION ( 'NONE',  ( 0.000000000000000000, -0.000000000000000000, 1.000000000000000000 ) ) ;
#44981=DIRECTION ( 'NONE',  ( 3.469446951953631938E-15, 1.000000000000000000, 0.000000000000000000 ) ) ;
#45012=ORIENTED_EDGE ( 'NONE', *, *, #25988, .T. ) ;
#45082=ORIENTED_EDGE ( 'NONE', *, *, #19218, .F. ) ;
#45083=CARTESIAN_POINT ( 'NONE',  ( -7.957671378281915615E-17, 0.1564960629921311464, -0.3937007874015748254 ) ) ;
#45116=DIRECTION ( 'NONE',  ( 1.000000000000000000, -3.469446951953626022E-15, -0.000000000000000000 ) ) ;
#45148=AXIS2_PLACEMENT_3D ( 'NONE', #31336, #9523, #12891 ) ;
#45227=ORIENTED_EDGE ( 'NONE', *, *, #43590, .T. ) ;
#45353=COLOUR_RGB ( '', 0.09019608, 0.27058824, 0.51372549) ;
#45382=CARTESIAN_POINT ( 'NONE',  ( 0.5555748031496083872, 0.1864803149606324151, 0.01858545845903139190 ) ) ;
#45389=EDGE_CURVE ( 'NONE', #33534, #16814, #23067, .T. ) ;
#45418=LINE ( 'NONE', #47444, #3897 ) ;
#45498=CARTESIAN_POINT ( 'NONE',  ( 0.3980944881889786346, 0.6449983665207558170, -0.7480314960629921295 ) ) ;
#45539=AXIS2_PLACEMENT_3D ( 'NONE', #35111, #38455, #31285 ) ;
#45567=CIRCLE ( 'NONE', #11183, 0.1864803149606298893 ) ;
#45596=CARTESIAN_POINT ( 'NONE',  ( 0.5555748031496099415, 0.6449983665207552619, -0.06082000038405668829 ) ) ;
#45607=VECTOR ( 'NONE', #35096, 39.37007874015748143 ) ;
#45628=ORIENTED_EDGE ( 'NONE', *, *, #39100, .F. ) ;
#45786=ADVANCED_FACE ( 'NONE', ( #2727 ), #9714, .F. ) ;
#45799=EDGE_LOOP ( 'NONE', ( #45012, #931, #26203, #22478 ) ) ;
#45838=CYLINDRICAL_SURFACE ( 'NONE', #47017, 0.6872114956789353579 ) ;
#45869=EDGE_CURVE ( 'NONE', #157, #30455, #38707, .T. ) ;
#45871=ORIENTED_EDGE ( 'NONE', *, *, #12795, .T. ) ;
#45874=PLANE ( 'NONE',  #27692 ) ;
#45875=ADVANCED_FACE ( 'NONE', ( #13763 ), #45874, .F. ) ;
#46003=AXIS2_PLACEMENT_3D ( 'NONE', #43285, #25581, #22423 ) ;
#46091=PRODUCT_DEFINITION_CONTEXT ( 'detailed design', #38264, 'design' ) ;
#46111=AXIS2_PLACEMENT_3D ( 'NONE', #35199, #16740, #38780 ) ;
#46129=CIRCLE ( 'NONE', #29381, 0.6872114956789353579 ) ;
#46134=EDGE_LOOP ( 'NONE', ( #14945, #36932, #45227, #35038 ) ) ;
#46136=DIRECTION ( 'NONE',  ( 1.000000000000000000, -3.469446951953626022E-15, -0.000000000000000000 ) ) ;
#46241=EDGE_CURVE ( 'NONE', #10953, #1004, #15449, .T. ) ;
#46312=EDGE_LOOP ( 'NONE', ( #10480, #4360, #26445, #6360 ) ) ;
#46342=ORIENTED_EDGE ( 'NONE', *, *, #1198, .F. ) ;
#46344=CONICAL_SURFACE ( 'NONE', #45539, 0.1003937007874011050, 0.7853981633973787790 ) ;
#46368=DIRECTION ( 'NONE',  ( 1.000000000000000000, -3.469446951953613794E-15, 0.000000000000000000 ) ) ;
#46421=DIRECTION ( 'NONE',  ( -0.000000000000000000, 0.000000000000000000, -1.000000000000000000 ) ) ;
#46455=DIRECTION ( 'NONE',  ( 1.000000000000000000, -3.469446951953613794E-15, -0.000000000000000000 ) ) ;
#46571=EDGE_CURVE ( 'NONE', #21208, #33536, #13169, .T. ) ;
#46575=VERTEX_POINT ( 'NONE', #25455 ) ;
#46593=CARTESIAN_POINT ( 'NONE',  ( -0.3690944881889767215, 5.424056872940433071E-15, 0.7480314960629921295 ) ) ;
#46627=CIRCLE ( 'NONE', #3773, 0.1003937007874011050 ) ;
#46642=DIRECTION ( 'NONE',  ( -1.000000000000000000, 3.469446951953626022E-15, 0.000000000000000000 ) ) ;
#46707=CYLINDRICAL_SURFACE ( 'NONE', #12280, 0.1377952755905509086 ) ;
#46729=ORIENTED_EDGE ( 'NONE', *, *, #44244, .F. ) ;
#46859=ORIENTED_EDGE ( 'NONE', *, *, #15932, .F. ) ;
#46895=SURFACE_STYLE_USAGE ( .BOTH. , #35195 ) ;
#47017=AXIS2_PLACEMENT_3D ( 'NONE', #45596, #42864, #27683 ) ;
#47081=LINE ( 'NONE', #3478, #2094 ) ;
#47106=VECTOR ( 'NONE', #13702, 39.37007874015748143 ) ;
#47181=DIRECTION ( 'NONE',  ( 1.267059173938978811E-30, 3.652049423109077687E-16, -1.000000000000000000 ) ) ;
#47306=CARTESIAN_POINT ( 'NONE',  ( 0.5555748031496086092, 0.2597269656108935343, 0.5511811023622046335 ) ) ;
#47331=DIRECTION ( 'NONE',  ( 1.541976423090495042E-15, 0.4344452574044144755, -0.9006982393225890782 ) ) ;
#47444=CARTESIAN_POINT ( 'NONE',  ( 1.614954907737318939E-16, 0.1564960629921311464, 0.4940944881889759444 ) ) ;
ENDSEC;
END-ISO-10303-21;
